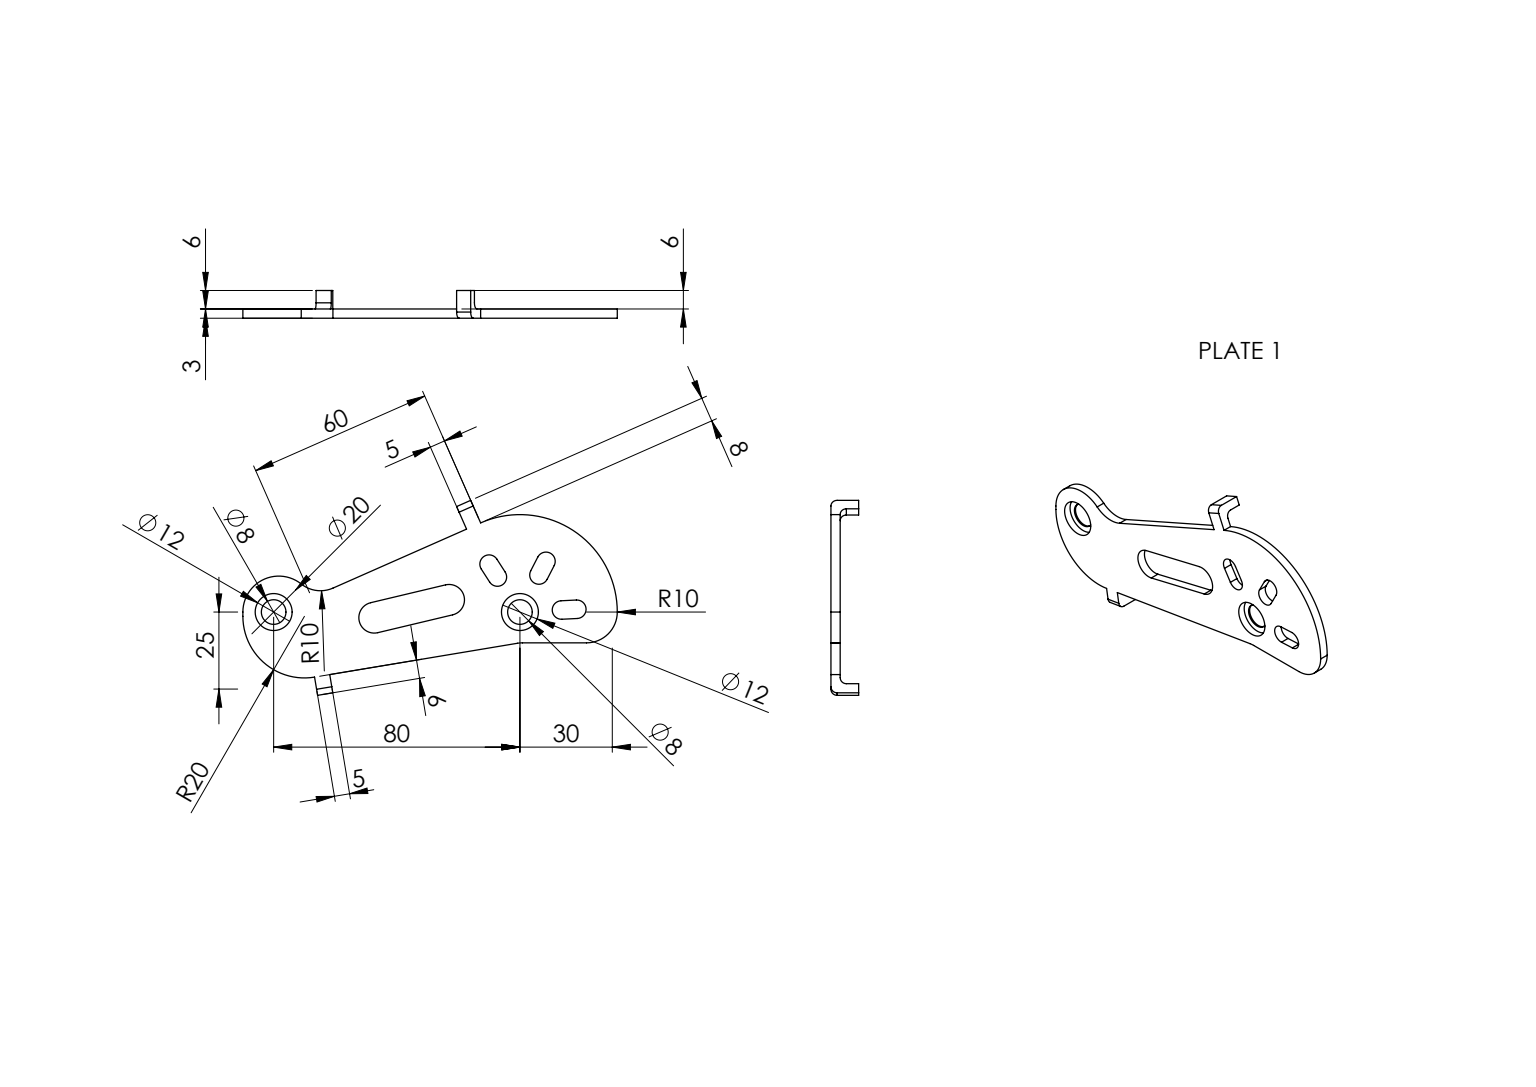
ISO-10303-21;
HEADER;
FILE_DESCRIPTION (('STEP AP214'),
    '1' );
FILE_NAME ('plate 1.step',
    '2026-10-31T03:41:51',
    ( '' ),
    ( '' ),
    'SwSTEP 2.0',
    'SolidWorks 2026',
    '' );
FILE_SCHEMA (( 'AUTOMOTIVE_DESIGN' ));
ENDSEC;

DATA;
#1=DIRECTION ( 'NONE',  ( 0.000000000000000000, 0.000000000000000000, 1.000000000000000000 ) ) ;
#5=CARTESIAN_POINT ( 'NONE',  ( 67.45386469005195806, 13.93318132202354676, 7.000000000000000000 ) ) ;
#9=ORIENTED_EDGE ( 'NONE', *, *, #4269, .F. ) ;
#17=DIRECTION ( 'NONE',  ( 1.000000000000000000, 0.000000000000000000, 0.000000000000000000 ) ) ;
#21=ORIENTED_EDGE ( 'NONE', *, *, #15147, .T. ) ;
#26=CARTESIAN_POINT ( 'NONE',  ( 101.4858053992934401, 0.9022481406819604643, 7.000000000000000000 ) ) ;
#27=DIRECTION ( 'NONE',  ( 1.000000000000000000, 0.000000000000000000, 0.000000000000000000 ) ) ;
#38=EDGE_LOOP ( 'NONE', ( #950, #5937 ) ) ;
#43=DIRECTION ( 'NONE',  ( -0.9863939238321437486, -0.1643989873053572359, 0.000000000000000000 ) ) ;
#44=CARTESIAN_POINT ( 'NONE',  ( 67.45386469005195806, 13.93318132202354676, 4.000000000000000000 ) ) ;
#50=ORIENTED_EDGE ( 'NONE', *, *, #12668, .F. ) ;
#54=ORIENTED_EDGE ( 'NONE', *, *, #8757, .F. ) ;
#57=DIRECTION ( 'NONE',  ( 0.9863939238321437486, 0.1643989873053572359, -0.000000000000000000 ) ) ;
#65=DIRECTION ( 'NONE',  ( 1.000000000000000000, 0.000000000000000000, 0.000000000000000000 ) ) ;
#76=ORIENTED_EDGE ( 'NONE', *, *, #9574, .F. ) ;
#100=CARTESIAN_POINT ( 'NONE',  ( 72.68384697807672978, 11.35494834827056110, 7.000000000000000000 ) ) ;
#101=DIRECTION ( 'NONE',  ( 0.000000000000000000, 0.000000000000000000, 1.000000000000000000 ) ) ;
#112=CYLINDRICAL_SURFACE ( 'NONE', #13936, 11.66666666666667318 ) ;
#118=CIRCLE ( 'NONE', #10455, 4.999999999999997335 ) ;
#128=EDGE_LOOP ( 'NONE', ( #4298, #9010, #776, #2710 ) ) ;
#137=CARTESIAN_POINT ( 'NONE',  ( 101.6227766016837819, 5.204170427930421283E-15, -130.1575142076926852 ) ) ;
#138=DIRECTION ( 'NONE',  ( -0.000000000000000000, -0.000000000000000000, 1.000000000000000000 ) ) ;
#151=DIRECTION ( 'NONE',  ( -0.8406209333187997235, -0.5416238976136763528, 0.000000000000000000 ) ) ;
#154=VERTEX_POINT ( 'NONE', #3488 ) ;
#169=DIRECTION ( 'NONE',  ( -0.9148936170212769170, -0.4036950204470262649, 0.000000000000000000 ) ) ;
#170=EDGE_CURVE ( 'NONE', #1510, #11203, #8177, .T. ) ;
#178=DIRECTION ( 'NONE',  ( 0.9148936170212770280, 0.4036950204470263204, -0.000000000000000000 ) ) ;
#179=DIRECTION ( 'NONE',  ( -0.9728364810787193395, -0.2314933715733012709, -0.000000000000000000 ) ) ;
#185=AXIS2_PLACEMENT_3D ( 'NONE', #6437, #12199, #1683 ) ;
#202=DIRECTION ( 'NONE',  ( -0.000000000000000000, -0.000000000000000000, -1.000000000000000000 ) ) ;
#209=VECTOR ( 'NONE', #6552, 1000.000000000000114 ) ;
#226=CIRCLE ( 'NONE', #8834, 6.000000000000005329 ) ;
#240=CARTESIAN_POINT ( 'NONE',  ( 0.000000000000000000, 0.000000000000000000, 4.500000000000000888 ) ) ;
#241=VERTEX_POINT ( 'NONE', #12080 ) ;
#257=EDGE_CURVE ( 'NONE', #8622, #3271, #11448, .T. ) ;
#261=DIRECTION ( 'NONE',  ( -2.081668171172168513E-16, 1.000000000000000000, 0.000000000000000000 ) ) ;
#265=EDGE_LOOP ( 'NONE', ( #1777, #5909, #7218, #13127 ) ) ;
#278=CYLINDRICAL_SURFACE ( 'NONE', #5273, 4.000000000000003553 ) ;
#279=ORIENTED_EDGE ( 'NONE', *, *, #14874, .F. ) ;
#287=EDGE_LOOP ( 'NONE', ( #9306, #900, #54, #10982, #12376 ) ) ;
#291=VECTOR ( 'NONE', #10020, 999.9999999999998863 ) ;
#292=VECTOR ( 'NONE', #261, 1000.000000000000000 ) ;
#303=ORIENTED_EDGE ( 'NONE', *, *, #14839, .T. ) ;
#307=LINE ( 'NONE', #10624, #1105 ) ;
#324=EDGE_LOOP ( 'NONE', ( #378, #14042, #4793, #7094 ) ) ;
#328=SURFACE_STYLE_USAGE ( .BOTH. , #10800 ) ;
#330=CIRCLE ( 'NONE', #3305, 2.999999999999988898 ) ;
#356=DIRECTION ( 'NONE',  ( 0.000000000000000000, -0.000000000000000000, -1.000000000000000000 ) ) ;
#363=ORIENTED_EDGE ( 'NONE', *, *, #14313, .F. ) ;
#370=DIRECTION ( 'NONE',  ( -0.000000000000000000, -0.000000000000000000, -1.000000000000000000 ) ) ;
#378=ORIENTED_EDGE ( 'NONE', *, *, #2401, .F. ) ;
#380=VECTOR ( 'NONE', #3922, 1000.000000000000000 ) ;
#414=VECTOR ( 'NONE', #3445, 1000.000000000000114 ) ;
#437=EDGE_CURVE ( 'NONE', #12266, #2494, #3436, .T. ) ;
#449=CARTESIAN_POINT ( 'NONE',  ( 4.000000000000000000, 4.898587196589412829E-16, 7.000000000000000000 ) ) ;
#459=CIRCLE ( 'NONE', #717, 20.00000000000000000 ) ;
#478=LINE ( 'NONE', #13313, #9423 ) ;
#497=VERTEX_POINT ( 'NONE', #5831 ) ;
#514=CARTESIAN_POINT ( 'NONE',  ( 75.20570977803312473, 12.97982004111160315, 7.000000000000000000 ) ) ;
#564=CARTESIAN_POINT ( 'NONE',  ( 101.6227766016837819, -9.999999999999994671, 4.000000000000003553 ) ) ;
#582=CARTESIAN_POINT ( 'NONE',  ( 80.00000000000000000, -9.999999999999994671, -130.1575142076926852 ) ) ;
#585=CARTESIAN_POINT ( 'NONE',  ( 83.50748565343083385, 13.38500995229612478, 7.000000000000000000 ) ) ;
#593=ADVANCED_FACE ( 'NONE', ( #8410 ), #2741, .F. ) ;
#611=DIRECTION ( 'NONE',  ( 0.9863939238321437486, 0.1643989873053572359, -0.000000000000000000 ) ) ;
#613=VERTEX_POINT ( 'NONE', #6348 ) ;
#618=ORIENTED_EDGE ( 'NONE', *, *, #1784, .F. ) ;
#619=ORIENTED_EDGE ( 'NONE', *, *, #14712, .T. ) ;
#652=DIRECTION ( 'NONE',  ( 0.9148936170212769170, 0.4036950204470262649, 0.000000000000000000 ) ) ;
#657=DIRECTION ( 'NONE',  ( -0.000000000000000000, -0.000000000000000000, -1.000000000000000000 ) ) ;
#662=ORIENTED_EDGE ( 'NONE', *, *, #2587, .T. ) ;
#665=DIRECTION ( 'NONE',  ( 0.000000000000000000, 0.000000000000000000, 1.000000000000000000 ) ) ;
#674=LINE ( 'NONE', #9057, #4725 ) ;
#693=LINE ( 'NONE', #9146, #14795 ) ;
#700=ORIENTED_EDGE ( 'NONE', *, *, #12767, .F. ) ;
#710=LINE ( 'NONE', #10011, #13396 ) ;
#715=LINE ( 'NONE', #4102, #2549 ) ;
#717=AXIS2_PLACEMENT_3D ( 'NONE', #10345, #13964, #27 ) ;
#731=EDGE_LOOP ( 'NONE', ( #12337, #9873, #12437, #11706, #9637 ) ) ;
#744=FACE_OUTER_BOUND ( 'NONE', #8998, .T. ) ;
#753=EDGE_LOOP ( 'NONE', ( #1969, #1811, #5274, #1615 ) ) ;
#758=ORIENTED_EDGE ( 'NONE', *, *, #5172, .T. ) ;
#769=DIRECTION ( 'NONE',  ( -0.9863939238321437486, -0.1643989873053574857, 0.000000000000000000 ) ) ;
#774=ORIENTED_EDGE ( 'NONE', *, *, #12921, .T. ) ;
#776=ORIENTED_EDGE ( 'NONE', *, *, #5121, .F. ) ;
#785=AXIS2_PLACEMENT_3D ( 'NONE', #4746, #10427, #14110 ) ;
#800=CARTESIAN_POINT ( 'NONE',  ( 59.43001430450886602, 34.23215029930534570, -8.169391093593850073 ) ) ;
#818=ORIENTED_EDGE ( 'NONE', *, *, #10308, .T. ) ;
#825=ORIENTED_EDGE ( 'NONE', *, *, #12060, .T. ) ;
#845=VECTOR ( 'NONE', #12005, 1000.000000000000000 ) ;
#846=VECTOR ( 'NONE', #7852, 1000.000000000000000 ) ;
#857=ADVANCED_FACE ( 'NONE', ( #3913 ), #278, .F. ) ;
#872=VECTOR ( 'NONE', #5496, 1000.000000000000000 ) ;
#873=DIRECTION ( 'NONE',  ( 0.1643989873053570416, -0.9863939238321438596, 0.000000000000000000 ) ) ;
#900=ORIENTED_EDGE ( 'NONE', *, *, #3910, .F. ) ;
#901=EDGE_CURVE ( 'NONE', #14849, #9696, #2754, .T. ) ;
#915=EDGE_CURVE ( 'NONE', #3460, #13819, #8735, .T. ) ;
#919=CARTESIAN_POINT ( 'NONE',  ( 72.68384697807672978, 11.35494834827056110, -2.000000000000000888 ) ) ;
#924=CIRCLE ( 'NONE', #3389, 2.000000000000003109 ) ;
#927=ORIENTED_EDGE ( 'NONE', *, *, #12743, .T. ) ;
#948=CARTESIAN_POINT ( 'NONE',  ( 67.23404255319148604, 28.93147646537027384, -130.1575142076926852 ) ) ;
#950=ORIENTED_EDGE ( 'NONE', *, *, #6665, .T. ) ;
#974=ORIENTED_EDGE ( 'NONE', *, *, #2510, .F. ) ;
#975=CARTESIAN_POINT ( 'NONE',  ( 31.51081190520435626, 3.030430839836910639, 4.000000000000000000 ) ) ;
#1017=SHAPE_REPRESENTATION ( 'plate 1', ( #1376 ), #2887 ) ;
#1020=EDGE_CURVE ( 'NONE', #4343, #12388, #6600, .T. ) ;
#1023=CARTESIAN_POINT ( 'NONE',  ( 10.00000000000000178, -1.390791565672601315, -130.1575142076926852 ) ) ;
#1024=PLANE ( 'NONE',  #2586 ) ;
#1043=CARTESIAN_POINT ( 'NONE',  ( 59.43001430450886602, 34.23215029930534570, -2.000000000000000000 ) ) ;
#1060=EDGE_LOOP ( 'NONE', ( #3025, #4253, #9240, #3645 ) ) ;
#1084=DIRECTION ( 'NONE',  ( 0.000000000000000000, 0.000000000000000000, 1.000000000000000000 ) ) ;
#1090=CARTESIAN_POINT ( 'NONE',  ( 33.82574562093736859, -6.697933970950280091, 7.000000000000000000 ) ) ;
#1093=EDGE_CURVE ( 'NONE', #6683, #14792, #3780, .T. ) ;
#1105=VECTOR ( 'NONE', #3625, 1000.000000000000000 ) ;
#1115=AXIS2_PLACEMENT_3D ( 'NONE', #3624, #4719, #10846 ) ;
#1127=CARTESIAN_POINT ( 'NONE',  ( 80.00000000000000000, 0.000000000000000000, 4.500000000000000888 ) ) ;
#1131=LINE ( 'NONE', #9501, #6687 ) ;
#1137=CIRCLE ( 'NONE', #7021, 3.000000000000002665 ) ;
#1142=CARTESIAN_POINT ( 'NONE',  ( 1.666666666666673624, 0.000000000000000000, -130.1575142076926852 ) ) ;
#1147=DIRECTION ( 'NONE',  ( 1.000000000000000000, 0.000000000000000000, 0.000000000000000000 ) ) ;
#1159=ORIENTED_EDGE ( 'NONE', *, *, #1020, .T. ) ;
#1166=CIRCLE ( 'NONE', #11222, 10.00000000000000000 ) ;
#1168=CIRCLE ( 'NONE', #14164, 9.999999999999994671 ) ;
#1179=ADVANCED_FACE ( 'NONE', ( #3555 ), #5032, .F. ) ;
#1181=VERTEX_POINT ( 'NONE', #1182 ) ;
#1182=CARTESIAN_POINT ( 'NONE',  ( 76.00000000000000000, 4.898587196589422689E-16, 4.500000000000003553 ) ) ;
#1191=CARTESIAN_POINT ( 'NONE',  ( 111.6227766016837961, 7.610970684806392799E-15, -130.1575142076926852 ) ) ;
#1192=CARTESIAN_POINT ( 'NONE',  ( 101.4858053992934401, 0.9022481406819604643, -2.000000000000000888 ) ) ;
#1193=ORIENTED_EDGE ( 'NONE', *, *, #15025, .F. ) ;
#1199=DIRECTION ( 'NONE',  ( -0.000000000000000000, -0.000000000000000000, 1.000000000000000000 ) ) ;
#1202=VECTOR ( 'NONE', #1786, 1000.000000000000000 ) ;
#1208=CARTESIAN_POINT ( 'NONE',  ( 88.84370878116858705, 10.64188714589527507, 7.000000000000000000 ) ) ;
#1223=EDGE_CURVE ( 'NONE', #8917, #4042, #1637, .T. ) ;
#1230=LINE ( 'NONE', #5986, #13850 ) ;
#1238=CYLINDRICAL_SURFACE ( 'NONE', #11480, 9.999999999999994671 ) ;
#1240=FACE_OUTER_BOUND ( 'NONE', #4768, .T. ) ;
#1244=ORIENTED_EDGE ( 'NONE', *, *, #9119, .F. ) ;
#1245=DIRECTION ( 'NONE',  ( -0.9863939238321437486, -0.1643989873053572359, 0.000000000000000000 ) ) ;
#1268=FACE_OUTER_BOUND ( 'NONE', #5575, .T. ) ;
#1281=CARTESIAN_POINT ( 'NONE',  ( 101.6227766016837819, -9.999999999999994671, 7.000000000000000000 ) ) ;
#1301=DIRECTION ( 'NONE',  ( -0.9863939238321436376, -0.1643989873053573192, 0.000000000000000000 ) ) ;
#1302=DIRECTION ( 'NONE',  ( -0.9863939238321437486, -0.1643989873053574857, 0.000000000000000000 ) ) ;
#1309=DIRECTION ( 'NONE',  ( 0.000000000000000000, 0.000000000000000000, 1.000000000000000000 ) ) ;
#1319=CARTESIAN_POINT ( 'NONE',  ( 19.20634328910001543, -26.21503864878155099, 4.000000000000000000 ) ) ;
#1320=ORIENTED_EDGE ( 'NONE', *, *, #13609, .F. ) ;
#1326=CIRCLE ( 'NONE', #12616, 31.62277660168379256 ) ;
#1328=ORIENTED_EDGE ( 'NONE', *, *, #3928, .F. ) ;
#1332=DIRECTION ( 'NONE',  ( -0.000000000000000000, -0.000000000000000000, 1.000000000000000000 ) ) ;
#1335=CARTESIAN_POINT ( 'NONE',  ( 80.00000000000000000, 0.000000000000000000, 4.500000000000000888 ) ) ;
#1342=DIRECTION ( 'NONE',  ( -0.000000000000000000, -0.000000000000000000, 1.000000000000000000 ) ) ;
#1353=CIRCLE ( 'NONE', #6761, 4.000000000000000000 ) ;
#1354=ORIENTED_EDGE ( 'NONE', *, *, #15079, .F. ) ;
#1358=CARTESIAN_POINT ( 'NONE',  ( 88.84370878116858705, 10.64188714589527507, -2.000000000000000888 ) ) ;
#1367=EDGE_LOOP ( 'NONE', ( #7183, #13097, #9718, #13636 ) ) ;
#1376=AXIS2_PLACEMENT_3D ( 'NONE', #7353, #6187, #9640 ) ;
#1385=DIRECTION ( 'NONE',  ( 1.000000000000000000, 0.000000000000000000, 0.000000000000000000 ) ) ;
#1396=ORIENTED_EDGE ( 'NONE', *, *, #2874, .T. ) ;
#1401=ORIENTED_EDGE ( 'NONE', *, *, #5062, .F. ) ;
#1404=CIRCLE ( 'NONE', #13462, 4.000000000000000000 ) ;
#1412=DIRECTION ( 'NONE',  ( -0.9988110320138940956, -0.04874958797097371510, 0.000000000000000000 ) ) ;
#1418=VECTOR ( 'NONE', #11737, 1000.000000000000000 ) ;
#1424=DIRECTION ( 'NONE',  ( 1.000000000000000000, 0.000000000000000000, -0.000000000000000000 ) ) ;
#1428=LINE ( 'NONE', #8483, #6858 ) ;
#1440=VECTOR ( 'NONE', #1301, 1000.000000000000114 ) ;
#1445=CARTESIAN_POINT ( 'NONE',  ( 67.23404255319145761, 28.93147646537025963, 7.000000000000000000 ) ) ;
#1452=EDGE_LOOP ( 'NONE', ( #12989, #5324, #2411, #6833, #11094 ) ) ;
#1459=EDGE_CURVE ( 'NONE', #9282, #1757, #10468, .T. ) ;
#1461=ORIENTED_EDGE ( 'NONE', *, *, #12060, .F. ) ;
#1463=ORIENTED_EDGE ( 'NONE', *, *, #915, .T. ) ;
#1468=DIRECTION ( 'NONE',  ( 0.000000000000000000, 0.000000000000000000, 1.000000000000000000 ) ) ;
#1474=ADVANCED_FACE ( 'NONE', ( #3181 ), #9091, .F. ) ;
#1475=EDGE_CURVE ( 'NONE', #7248, #11593, #5936, .T. ) ;
#1486=CARTESIAN_POINT ( 'NONE',  ( 80.00000000000000000, -9.999999999999994671, 7.000000000000000000 ) ) ;
#1489=EDGE_CURVE ( 'NONE', #12388, #13917, #12187, .T. ) ;
#1493=DIRECTION ( 'NONE',  ( -0.4036950204470279302, 0.9148936170212763619, 0.000000000000000000 ) ) ;
#1499=FACE_OUTER_BOUND ( 'NONE', #2066, .T. ) ;
#1500=LINE ( 'NONE', #12168, #14620 ) ;
#1504=VERTEX_POINT ( 'NONE', #14151 ) ;
#1505=PLANE ( 'NONE',  #15194 ) ;
#1506=CARTESIAN_POINT ( 'NONE',  ( 13.94557569532858032, -25.06424573764405395, 5.000000000000000000 ) ) ;
#1510=VERTEX_POINT ( 'NONE', #11832 ) ;
#1512=ORIENTED_EDGE ( 'NONE', *, *, #2860, .T. ) ;
#1513=FACE_OUTER_BOUND ( 'NONE', #3682, .T. ) ;
#1519=VERTEX_POINT ( 'NONE', #5 ) ;
#1521=DIRECTION ( 'NONE',  ( 0.000000000000000000, 0.000000000000000000, 1.000000000000000000 ) ) ;
#1530=LINE ( 'NONE', #9835, #380 ) ;
#1533=EDGE_LOOP ( 'NONE', ( #3960, #14213, #11513, #14850 ) ) ;
#1538=LINE ( 'NONE', #4939, #7482 ) ;
#1568=CARTESIAN_POINT ( 'NONE',  ( 85.79342132543153809, 17.83186255874426962, 4.000000000000000000 ) ) ;
#1572=PRESENTATION_STYLE_ASSIGNMENT (( #328 ) ) ;
#1576=AXIS2_PLACEMENT_3D ( 'NONE', #10565, #9261, #17 ) ;
#1578=PLANE ( 'NONE',  #2664 ) ;
#1601=DIRECTION ( 'NONE',  ( 1.000000000000000000, 0.000000000000000000, 0.000000000000000000 ) ) ;
#1610=ORIENTED_EDGE ( 'NONE', *, *, #10529, .F. ) ;
#1615=ORIENTED_EDGE ( 'NONE', *, *, #12503, .F. ) ;
#1636=EDGE_LOOP ( 'NONE', ( #8758, #1159, #8999, #4436 ) ) ;
#1637=LINE ( 'NONE', #14555, #13858 ) ;
#1646=VECTOR ( 'NONE', #5740, 1000.000000000000114 ) ;
#1653=FACE_BOUND ( 'NONE', #6790, .T. ) ;
#1658=COLOUR_RGB ( '',0.8941176470588234615, 0.8941176470588234615, 0.8941176470588234615 ) ;
#1661=DIRECTION ( 'NONE',  ( 0.000000000000000000, 0.000000000000000000, 1.000000000000000000 ) ) ;
#1668=ORIENTED_EDGE ( 'NONE', *, *, #2242, .F. ) ;
#1678=FACE_OUTER_BOUND ( 'NONE', #14305, .T. ) ;
#1679=CARTESIAN_POINT ( 'NONE',  ( 62.65957446808508280, 26.91300136313512681, -8.169391093593850073 ) ) ;
#1683=DIRECTION ( 'NONE',  ( 1.000000000000000000, 0.000000000000000000, 0.000000000000000000 ) ) ;
#1692=ORIENTED_EDGE ( 'NONE', *, *, #1093, .F. ) ;
#1700=CARTESIAN_POINT ( 'NONE',  ( 84.00000000000000000, 0.000000000000000000, 4.500000000000003553 ) ) ;
#1701=AXIS2_PLACEMENT_3D ( 'NONE', #11946, #12178, #7362 ) ;
#1708=ORIENTED_EDGE ( 'NONE', *, *, #4189, .F. ) ;
#1709=AXIS2_PLACEMENT_3D ( 'NONE', #10548, #12901, #7081 ) ;
#1711=DIRECTION ( 'NONE',  ( 0.9988110320138940956, 0.04874958797097355551, -0.000000000000000000 ) ) ;
#1717=DIRECTION ( 'NONE',  ( 0.9988110320138940956, 0.04874958797097354857, 0.000000000000000000 ) ) ;
#1721=CARTESIAN_POINT ( 'NONE',  ( 98.63205416320636232, -2.094184955359725375, 7.000000000000000000 ) ) ;
#1735=ORIENTED_EDGE ( 'NONE', *, *, #3302, .F. ) ;
#1742=VERTEX_POINT ( 'NONE', #7398 ) ;
#1752=FACE_OUTER_BOUND ( 'NONE', #12919, .T. ) ;
#1757=VERTEX_POINT ( 'NONE', #1773 ) ;
#1758=EDGE_CURVE ( 'NONE', #6683, #11986, #9775, .T. ) ;
#1763=( NAMED_UNIT ( * ) PLANE_ANGLE_UNIT ( ) SI_UNIT ( $, .RADIAN. ) );
#1771=DIRECTION ( 'NONE',  ( 0.9148936170212769170, 0.4036950204470262649, -0.000000000000000000 ) ) ;
#1773=CARTESIAN_POINT ( 'NONE',  ( 19.25177984293775069, 7.759396820770414926, 7.000000000000000000 ) ) ;
#1774=PLANE ( 'NONE',  #6975 ) ;
#1777=ORIENTED_EDGE ( 'NONE', *, *, #7772, .F. ) ;
#1784=EDGE_CURVE ( 'NONE', #2017, #6698, #6767, .T. ) ;
#1786=DIRECTION ( 'NONE',  ( 0.9863939238321437486, 0.1643989873053572359, -0.000000000000000000 ) ) ;
#1792=DIRECTION ( 'NONE',  ( 0.000000000000000000, 0.000000000000000000, 1.000000000000000000 ) ) ;
#1807=CARTESIAN_POINT ( 'NONE',  ( 75.20570977803312473, 12.97982004111159959, 4.000000000000000000 ) ) ;
#1811=ORIENTED_EDGE ( 'NONE', *, *, #7772, .T. ) ;
#1833=APPLICATION_CONTEXT ( 'automotive_design' ) ;
#1851=CYLINDRICAL_SURFACE ( 'NONE', #15082, 2.999999999999988898 ) ;
#1861=VERTEX_POINT ( 'NONE', #15066 ) ;
#1872=LINE ( 'NONE', #4418, #7681 ) ;
#1886=VECTOR ( 'NONE', #7004, 1000.000000000000000 ) ;
#1900=VECTOR ( 'NONE', #3511, 1000.000000000000000 ) ;
#1916=EDGE_CURVE ( 'NONE', #9387, #10729, #2530, .T. ) ;
#1930=DIRECTION ( 'NONE',  ( -0.9988110320138940956, -0.04874958797097371510, 0.000000000000000000 ) ) ;
#1936=LINE ( 'NONE', #4397, #846 ) ;
#1956=ADVANCED_FACE ( 'NONE', ( #5922 ), #8208, .F. ) ;
#1969=ORIENTED_EDGE ( 'NONE', *, *, #5841, .F. ) ;
#1987=DIRECTION ( 'NONE',  ( -0.000000000000000000, -0.000000000000000000, 1.000000000000000000 ) ) ;
#1993=VERTEX_POINT ( 'NONE', #9369 ) ;
#2006=CARTESIAN_POINT ( 'NONE',  ( 67.23404255319145761, 28.93147646537026318, -130.1575142076926852 ) ) ;
#2017=VERTEX_POINT ( 'NONE', #8661 ) ;
#2019=CARTESIAN_POINT ( 'NONE',  ( 8.961831343790189308, 9.104486995144789319, 4.000000000000003553 ) ) ;
#2030=DIRECTION ( 'NONE',  ( -0.000000000000000000, -0.000000000000000000, 1.000000000000000000 ) ) ;
#2046=LINE ( 'NONE', #14745, #1646 ) ;
#2052=CARTESIAN_POINT ( 'NONE',  ( 61.98919079003883326, 3.953582723775848962, 4.000000000000000000 ) ) ;
#2057=PRODUCT_DEFINITION_FORMATION_WITH_SPECIFIED_SOURCE ( 'ANY', '', #2480, .NOT_KNOWN. ) ;
#2065=LINE ( 'NONE', #6682, #14927 ) ;
#2066=EDGE_LOOP ( 'NONE', ( #2156, #3607, #7181, #7620, #5886, #1396, #303, #3086, #8875, #8957, #1193, #6098, #2265, #14266, #3257, #5444 ) ) ;
#2072=CARTESIAN_POINT ( 'NONE',  ( 18.21994936526786901, -20.29667510578869027, 4.000000000000000000 ) ) ;
#2076=VECTOR ( 'NONE', #8244, 1000.000000000000000 ) ;
#2080=ORIENTED_EDGE ( 'NONE', *, *, #12668, .T. ) ;
#2098=ORIENTED_EDGE ( 'NONE', *, *, #9330, .T. ) ;
#2107=EDGE_CURVE ( 'NONE', #14957, #4472, #1137, .T. ) ;
#2110=EDGE_LOOP ( 'NONE', ( #7467, #6376, #974, #76 ) ) ;
#2115=ORIENTED_EDGE ( 'NONE', *, *, #1223, .F. ) ;
#2121=DIRECTION ( 'NONE',  ( 0.000000000000000000, 0.000000000000000000, 1.000000000000000000 ) ) ;
#2142=VECTOR ( 'NONE', #4991, 1000.000000000000114 ) ;
#2153=FACE_OUTER_BOUND ( 'NONE', #11801, .T. ) ;
#2156=ORIENTED_EDGE ( 'NONE', *, *, #7988, .F. ) ;
#2163=EDGE_CURVE ( 'NONE', #12183, #9373, #674, .T. ) ;
#2172=AXIS2_PLACEMENT_3D ( 'NONE', #13204, #5001, #5160 ) ;
#2173=CARTESIAN_POINT ( 'NONE',  ( 18.87754531448929995, -24.24225080111726527, 7.000000000000000000 ) ) ;
#2175=DIRECTION ( 'NONE',  ( -0.9148936170212765839, -0.4036950204470271530, 0.000000000000000000 ) ) ;
#2180=AXIS2_PLACEMENT_3D ( 'NONE', #13581, #14822, #3143 ) ;
#2182=DIRECTION ( 'NONE',  ( 1.000000000000000000, 0.000000000000000000, 0.000000000000000000 ) ) ;
#2183=DIRECTION ( 'NONE',  ( 0.8406209333187990573, 0.5416238976136774630, 0.000000000000000000 ) ) ;
#2186=DIRECTION ( 'NONE',  ( 1.000000000000000000, 0.000000000000000000, 0.000000000000000000 ) ) ;
#2194=LINE ( 'NONE', #14091, #10899 ) ;
#2204=EDGE_CURVE ( 'NONE', #4704, #4042, #8972, .T. ) ;
#2227=DIRECTION ( 'NONE',  ( 0.000000000000000000, 0.000000000000000000, 1.000000000000000000 ) ) ;
#2242=EDGE_CURVE ( 'NONE', #10729, #12348, #10059, .T. ) ;
#2253=CARTESIAN_POINT ( 'NONE',  ( 80.00000000000000000, 0.000000000000000000, 4.500000000000000888 ) ) ;
#2255=VERTEX_POINT ( 'NONE', #7968 ) ;
#2265=ORIENTED_EDGE ( 'NONE', *, *, #2575, .T. ) ;
#2282=VECTOR ( 'NONE', #169, 1000.000000000000114 ) ;
#2298=DIRECTION ( 'NONE',  ( 1.000000000000000000, 0.000000000000000000, 0.000000000000000000 ) ) ;
#2313=AXIS2_PLACEMENT_3D ( 'NONE', #4662, #2489, #5948 ) ;
#2335=ADVANCED_FACE ( 'NONE', ( #5901 ), #9415, .F. ) ;
#2338=ORIENTED_EDGE ( 'NONE', *, *, #3364, .T. ) ;
#2342=AXIS2_PLACEMENT_3D ( 'NONE', #1319, #8384, #9549 ) ;
#2351=PLANE ( 'NONE',  #11505 ) ;
#2357=DIRECTION ( 'NONE',  ( 0.4571871344001383619, 0.8893705212896307888, 0.000000000000000000 ) ) ;
#2366=FACE_OUTER_BOUND ( 'NONE', #7966, .T. ) ;
#2396=EDGE_CURVE ( 'NONE', #8331, #14360, #13297, .T. ) ;
#2401=EDGE_CURVE ( 'NONE', #14060, #1181, #1131, .T. ) ;
#2402=CIRCLE ( 'NONE', #14437, 6.000000000000005329 ) ;
#2411=ORIENTED_EDGE ( 'NONE', *, *, #8973, .T. ) ;
#2449=DIRECTION ( 'NONE',  ( 1.000000000000000000, 0.000000000000000000, 0.000000000000000000 ) ) ;
#2460=ORIENTED_EDGE ( 'NONE', *, *, #11205, .F. ) ;
#2463=CARTESIAN_POINT ( 'NONE',  ( 6.000000000000000888, 0.000000000000000000, 7.000000000000000000 ) ) ;
#2469=DIRECTION ( 'NONE',  ( -0.1643989873053570416, 0.9863939238321438596, 0.000000000000000000 ) ) ;
#2471=CARTESIAN_POINT ( 'NONE',  ( 13.28797974610715116, -21.11867004231547540, 4.000000000000000000 ) ) ;
#2480=PRODUCT ( 'plate 1', 'plate 1', '', ( #7597 ) ) ;
#2489=DIRECTION ( 'NONE',  ( 0.000000000000000000, 0.000000000000000000, 1.000000000000000000 ) ) ;
#2493=ORIENTED_EDGE ( 'NONE', *, *, #4742, .F. ) ;
#2494=VERTEX_POINT ( 'NONE', #9875 ) ;
#2498=VECTOR ( 'NONE', #6820, 1000.000000000000000 ) ;
#2503=DIRECTION ( 'NONE',  ( -0.9863939238321437486, -0.1643989873053572359, 0.000000000000000000 ) ) ;
#2510=EDGE_CURVE ( 'NONE', #1861, #4961, #11576, .T. ) ;
#2521=DIRECTION ( 'NONE',  ( -0.9863939238321437486, -0.1643989873053572359, 0.000000000000000000 ) ) ;
#2530=LINE ( 'NONE', #13990, #14147 ) ;
#2539=DIRECTION ( 'NONE',  ( 1.000000000000000000, 0.000000000000000000, 0.000000000000000000 ) ) ;
#2548=VERTEX_POINT ( 'NONE', #564 ) ;
#2549=VECTOR ( 'NONE', #13472, 999.9999999999998863 ) ;
#2551=CIRCLE ( 'NONE', #4040, 3.000000000000002665 ) ;
#2557=CARTESIAN_POINT ( 'NONE',  ( 18.21994936526786901, -20.29667510578869027, 4.000000000000000000 ) ) ;
#2559=AXIS2_PLACEMENT_3D ( 'NONE', #8822, #6441, #9832 ) ;
#2562=ADVANCED_FACE ( 'NONE', ( #13330 ), #6268, .F. ) ;
#2573=CARTESIAN_POINT ( 'NONE',  ( 13.45237873341251067, -22.10506396614762537, 4.000000000000000000 ) ) ;
#2575=EDGE_CURVE ( 'NONE', #4314, #154, #2808, .T. ) ;
#2577=EDGE_CURVE ( 'NONE', #11593, #4343, #3734, .T. ) ;
#2584=VECTOR ( 'NONE', #1245, 1000.000000000000000 ) ;
#2586=AXIS2_PLACEMENT_3D ( 'NONE', #948, #4567, #6788 ) ;
#2587=EDGE_CURVE ( 'NONE', #6626, #2812, #9144, .T. ) ;
#2589=EDGE_LOOP ( 'NONE', ( #11388, #9055, #927, #8161 ) ) ;
#2590=VERTEX_POINT ( 'NONE', #1807 ) ;
#2593=CARTESIAN_POINT ( 'NONE',  ( 18.71314632718394222, -23.25585687728512241, -2.000000000000000000 ) ) ;
#2619=DIRECTION ( 'NONE',  ( 0.000000000000000000, 0.000000000000000000, 1.000000000000000000 ) ) ;
#2625=CIRCLE ( 'NONE', #6053, 1.999999999999998446 ) ;
#2631=ORIENTED_EDGE ( 'NONE', *, *, #5544, .T. ) ;
#2633=CARTESIAN_POINT ( 'NONE',  ( 70.16198417812034904, 9.730076655429538590, -2.000000000000000888 ) ) ;
#2636=ORIENTED_EDGE ( 'NONE', *, *, #2950, .F. ) ;
#2637=VECTOR ( 'NONE', #2746, 1000.000000000000000 ) ;
#2646=DIRECTION ( 'NONE',  ( 1.000000000000000000, 0.000000000000000000, 0.000000000000000000 ) ) ;
#2649=VECTOR ( 'NONE', #1199, 1000.000000000000000 ) ;
#2656=VERTEX_POINT ( 'NONE', #2964 ) ;
#2664=AXIS2_PLACEMENT_3D ( 'NONE', #12025, #5138, #7360 ) ;
#2667=PLANE ( 'NONE',  #12480 ) ;
#2668=DIRECTION ( 'NONE',  ( -1.000000000000000000, 0.000000000000000000, 0.000000000000000000 ) ) ;
#2674=ORIENTED_EDGE ( 'NONE', *, *, #1475, .F. ) ;
#2705=ORIENTED_EDGE ( 'NONE', *, *, #13390, .T. ) ;
#2709=EDGE_LOOP ( 'NONE', ( #3455, #2098 ) ) ;
#2710=ORIENTED_EDGE ( 'NONE', *, *, #12921, .F. ) ;
#2716=PRODUCT_DEFINITION_CONTEXT ( 'detailed design', #5486, 'design' ) ;
#2718=ORIENTED_EDGE ( 'NONE', *, *, #7125, .T. ) ;
#2723=LINE ( 'NONE', #2557, #9179 ) ;
#2726=EDGE_CURVE ( 'NONE', #11269, #13370, #10366, .T. ) ;
#2733=CARTESIAN_POINT ( 'NONE',  ( 0.000000000000000000, 0.000000000000000000, 7.000000000000000000 ) ) ;
#2736=CARTESIAN_POINT ( 'NONE',  ( 88.46153288930041469, 16.46030115554384565, 4.000000000000000000 ) ) ;
#2741=CYLINDRICAL_SURFACE ( 'NONE', #1701, 2.999999999999975131 ) ;
#2746=DIRECTION ( 'NONE',  ( 0.000000000000000000, 0.000000000000000000, 1.000000000000000000 ) ) ;
#2748=LINE ( 'NONE', #13340, #9757 ) ;
#2749=DIRECTION ( 'NONE',  ( -0.000000000000000000, -0.000000000000000000, 1.000000000000000000 ) ) ;
#2754=LINE ( 'NONE', #10969, #6483 ) ;
#2760=ORIENTED_EDGE ( 'NONE', *, *, #14481, .T. ) ;
#2776=EDGE_CURVE ( 'NONE', #8684, #11326, #11860, .T. ) ;
#2780=ORIENTED_EDGE ( 'NONE', *, *, #2726, .T. ) ;
#2799=EDGE_CURVE ( 'NONE', #5498, #1181, #8198, .T. ) ;
#2808=LINE ( 'NONE', #12175, #292 ) ;
#2812=VERTEX_POINT ( 'NONE', #12847 ) ;
#2817=VERTEX_POINT ( 'NONE', #12709 ) ;
#2835=DIRECTION ( 'NONE',  ( 0.5416238976136762417, -0.8406209333187996124, 0.000000000000000000 ) ) ;
#2860=EDGE_CURVE ( 'NONE', #11203, #4549, #10404, .T. ) ;
#2871=EDGE_LOOP ( 'NONE', ( #3029, #1463, #9846, #14579 ) ) ;
#2872=AXIS2_PLACEMENT_3D ( 'NONE', #1358, #14205, #14123 ) ;
#2874=EDGE_CURVE ( 'NONE', #2548, #11986, #2194, .T. ) ;
#2882=( NAMED_UNIT ( * ) SI_UNIT ( $, .STERADIAN. ) SOLID_ANGLE_UNIT ( ) );
#2883=DIRECTION ( 'NONE',  ( 0.000000000000000000, 0.000000000000000000, 1.000000000000000000 ) ) ;
#2887=( GEOMETRIC_REPRESENTATION_CONTEXT ( 3 ) GLOBAL_UNCERTAINTY_ASSIGNED_CONTEXT ( ( #8762 ) ) GLOBAL_UNIT_ASSIGNED_CONTEXT ( ( #5206, #8711, #2882 ) ) REPRESENTATION_CONTEXT ( 'NONE', 'WORKASPACE' ) );
#2892=VECTOR ( 'NONE', #14504, 1000.000000000000000 ) ;
#2896=ORIENTED_EDGE ( 'NONE', *, *, #14272, .T. ) ;
#2919=ADVANCED_FACE ( 'NONE', ( #9558 ), #1851, .F. ) ;
#2920=CARTESIAN_POINT ( 'NONE',  ( -4.000000000000000000, 0.000000000000000000, 4.500000000000000888 ) ) ;
#2930=CARTESIAN_POINT ( 'NONE',  ( 64.00448238961524794, 36.25062540154047497, 5.000000000000000888 ) ) ;
#2942=CARTESIAN_POINT ( 'NONE',  ( 19.20634328910001543, -26.21503864878155099, -2.000000000000000000 ) ) ;
#2949=CARTESIAN_POINT ( 'NONE',  ( 84.00000000000000000, 0.000000000000000000, 4.000000000000003553 ) ) ;
#2950=EDGE_CURVE ( 'NONE', #4042, #11203, #2551, .T. ) ;
#2964=CARTESIAN_POINT ( 'NONE',  ( 59.43001430450886602, 34.23215029930534570, 5.000000000000000888 ) ) ;
#2967=EDGE_CURVE ( 'NONE', #11474, #10155, #7711, .T. ) ;
#2969=ORIENTED_EDGE ( 'NONE', *, *, #2776, .F. ) ;
#2972=DIRECTION ( 'NONE',  ( 0.1643989873053574302, -0.9863939238321437486, 0.000000000000000000 ) ) ;
#2980=ADVANCED_FACE ( 'NONE', ( #3004 ), #1774, .F. ) ;
#2992=CARTESIAN_POINT ( 'NONE',  ( 6.000000000000000888, 0.000000000000000000, 4.500000000000000888 ) ) ;
#2998=EDGE_CURVE ( 'NONE', #4961, #5235, #11224, .T. ) ;
#3004=FACE_OUTER_BOUND ( 'NONE', #3852, .T. ) ;
#3016=LINE ( 'NONE', #2942, #5641 ) ;
#3022=DIRECTION ( 'NONE',  ( 0.000000000000000000, 0.000000000000000000, 1.000000000000000000 ) ) ;
#3025=ORIENTED_EDGE ( 'NONE', *, *, #3209, .T. ) ;
#3028=EDGE_LOOP ( 'NONE', ( #10679, #15182, #11673, #9697 ) ) ;
#3029=ORIENTED_EDGE ( 'NONE', *, *, #8709, .F. ) ;
#3030=CARTESIAN_POINT ( 'NONE',  ( 88.46153288930041469, 16.46030115554384565, 7.000000000000000000 ) ) ;
#3038=DIRECTION ( 'NONE',  ( 0.4036950204470263204, -0.9148936170212770280, 0.000000000000000000 ) ) ;
#3040=ORIENTED_EDGE ( 'NONE', *, *, #2967, .T. ) ;
#3041=DIRECTION ( 'NONE',  ( 0.5416238976136762417, -0.8406209333187997235, -0.000000000000000000 ) ) ;
#3048=ADVANCED_FACE ( 'NONE', ( #13603 ), #3085, .F. ) ;
#3085=CYLINDRICAL_SURFACE ( 'NONE', #9180, 6.000000000000000888 ) ;
#3086=ORIENTED_EDGE ( 'NONE', *, *, #9173, .T. ) ;
#3097=EDGE_CURVE ( 'NONE', #9387, #12669, #1936, .T. ) ;
#3104=CARTESIAN_POINT ( 'NONE',  ( 86.17559721729969624, 12.01344854909570259, 4.000000000000000000 ) ) ;
#3108=CARTESIAN_POINT ( 'NONE',  ( 93.34550147531103903, 3.654933296868752457, -2.000000000000000888 ) ) ;
#3124=DIRECTION ( 'NONE',  ( 0.1643989873053578465, -0.9863939238321436376, 0.000000000000000000 ) ) ;
#3143=DIRECTION ( 'NONE',  ( -0.4571871344001417481, -0.8893705212896291235, 0.000000000000000000 ) ) ;
#3164=ORIENTED_EDGE ( 'NONE', *, *, #9841, .T. ) ;
#3172=VERTEX_POINT ( 'NONE', #7995 ) ;
#3181=FACE_OUTER_BOUND ( 'NONE', #5045, .T. ) ;
#3209=EDGE_CURVE ( 'NONE', #4384, #13626, #1230, .T. ) ;
#3221=CARTESIAN_POINT ( 'NONE',  ( 74.00000000000000000, 7.347880794884117764E-16, 4.500000000000000888 ) ) ;
#3222=ORIENTED_EDGE ( 'NONE', *, *, #10042, .T. ) ;
#3242=VERTEX_POINT ( 'NONE', #2463 ) ;
#3249=ORIENTED_EDGE ( 'NONE', *, *, #10369, .F. ) ;
#3255=DIRECTION ( 'NONE',  ( -1.000000000000000000, 0.000000000000000000, 0.000000000000000000 ) ) ;
#3256=CARTESIAN_POINT ( 'NONE',  ( 69.97572749000833880, 15.55805301486455683, 7.000000000000000000 ) ) ;
#3257=ORIENTED_EDGE ( 'NONE', *, *, #13814, .T. ) ;
#3261=EDGE_CURVE ( 'NONE', #1993, #8917, #12384, .T. ) ;
#3271=VERTEX_POINT ( 'NONE', #10537 ) ;
#3272=CARTESIAN_POINT ( 'NONE',  ( 61.98919079003883326, 3.953582723775848962, 7.000000000000000000 ) ) ;
#3273=DIRECTION ( 'NONE',  ( 0.4036950204470283188, -0.9148936170212761398, -0.000000000000000000 ) ) ;
#3290=ORIENTED_EDGE ( 'NONE', *, *, #7125, .F. ) ;
#3292=VERTEX_POINT ( 'NONE', #12818 ) ;
#3294=CARTESIAN_POINT ( 'NONE',  ( 80.00000000000000000, 0.000000000000000000, 4.500000000000003553 ) ) ;
#3300=CARTESIAN_POINT ( 'NONE',  ( 66.02295749185037721, 31.67615731643408949, 4.000000000000000000 ) ) ;
#3302=EDGE_CURVE ( 'NONE', #3709, #8012, #6990, .T. ) ;
#3305=AXIS2_PLACEMENT_3D ( 'NONE', #3104, #1792, #11316 ) ;
#3330=DIRECTION ( 'NONE',  ( 0.000000000000000000, 0.000000000000000000, 1.000000000000000000 ) ) ;
#3334=FACE_OUTER_BOUND ( 'NONE', #753, .T. ) ;
#3352=DIRECTION ( 'NONE',  ( -0.4036950204470285408, 0.9148936170212760288, 0.000000000000000000 ) ) ;
#3364=EDGE_CURVE ( 'NONE', #8684, #5234, #9894, .T. ) ;
#3365=EDGE_CURVE ( 'NONE', #2017, #7876, #9196, .T. ) ;
#3368=CARTESIAN_POINT ( 'NONE',  ( 58.14665764790533586, -0.9105996816177489572, 7.000000000000000000 ) ) ;
#3370=ORIENTED_EDGE ( 'NONE', *, *, #8629, .T. ) ;
#3371=CIRCLE ( 'NONE', #11691, 3.000000000000002665 ) ;
#3389=AXIS2_PLACEMENT_3D ( 'NONE', #4691, #10814, #4989 ) ;
#3399=DIRECTION ( 'NONE',  ( 1.000000000000000000, 0.000000000000000000, 0.000000000000000000 ) ) ;
#3400=DIRECTION ( 'NONE',  ( 1.000000000000000000, 0.000000000000000000, 0.000000000000000000 ) ) ;
#3408=FACE_OUTER_BOUND ( 'NONE', #9800, .T. ) ;
#3409=DIRECTION ( 'NONE',  ( 0.000000000000000000, 0.000000000000000000, 1.000000000000000000 ) ) ;
#3413=CARTESIAN_POINT ( 'NONE',  ( 80.00000000000000000, 0.000000000000000000, -130.1575142076926852 ) ) ;
#3425=CARTESIAN_POINT ( 'NONE',  ( 66.02295749185039142, 31.67615731643408949, 2.000000000000000000 ) ) ;
#3433=ORIENTED_EDGE ( 'NONE', *, *, #5924, .T. ) ;
#3436=LINE ( 'NONE', #1208, #3855 ) ;
#3444=CARTESIAN_POINT ( 'NONE',  ( 59.43001430450886602, 34.23215029930534570, -8.169391093593850073 ) ) ;
#3445=DIRECTION ( 'NONE',  ( -0.5416238976136773520, 0.8406209333187989463, 0.000000000000000000 ) ) ;
#3448=DIRECTION ( 'NONE',  ( -0.000000000000000000, -0.000000000000000000, 1.000000000000000000 ) ) ;
#3455=ORIENTED_EDGE ( 'NONE', *, *, #15119, .T. ) ;
#3460=VERTEX_POINT ( 'NONE', #3221 ) ;
#3461=VERTEX_POINT ( 'NONE', #12516 ) ;
#3465=DIRECTION ( 'NONE',  ( 0.9988110320138940956, 0.04874958797097355551, 0.000000000000000000 ) ) ;
#3488=CARTESIAN_POINT ( 'NONE',  ( -9.999999999999998224, 0.000000000000000000, 4.000000000000003553 ) ) ;
#3494=CARTESIAN_POINT ( 'NONE',  ( 65.21556745095632834, 33.50594455047664866, -2.000000000000000000 ) ) ;
#3495=DIRECTION ( 'NONE',  ( -0.000000000000000000, -0.000000000000000000, 1.000000000000000000 ) ) ;
#3503=VECTOR ( 'NONE', #13162, 1000.000000000000000 ) ;
#3507=VERTEX_POINT ( 'NONE', #5529 ) ;
#3511=DIRECTION ( 'NONE',  ( 0.000000000000000000, 0.000000000000000000, 1.000000000000000000 ) ) ;
#3523=CARTESIAN_POINT ( 'NONE',  ( 67.23404255319148604, 28.93147646537027384, 4.000000000000003553 ) ) ;
#3525=EDGE_CURVE ( 'NONE', #3993, #3242, #3858, .T. ) ;
#3526=ORIENTED_EDGE ( 'NONE', *, *, #15119, .F. ) ;
#3542=VECTOR ( 'NONE', #2175, 1000.000000000000000 ) ;
#3552=AXIS2_PLACEMENT_3D ( 'NONE', #3800, #13014, #10801 ) ;
#3555=FACE_OUTER_BOUND ( 'NONE', #12397, .T. ) ;
#3560=DIRECTION ( 'NONE',  ( -1.000000000000000000, 0.000000000000000000, 0.000000000000000000 ) ) ;
#3561=ORIENTED_EDGE ( 'NONE', *, *, #15147, .F. ) ;
#3568=ORIENTED_EDGE ( 'NONE', *, *, #4269, .T. ) ;
#3570=CARTESIAN_POINT ( 'NONE',  ( 31.51081190520435626, 3.030430839836910639, 7.000000000000000000 ) ) ;
#3594=ORIENTED_EDGE ( 'NONE', *, *, #14695, .T. ) ;
#3607=ORIENTED_EDGE ( 'NONE', *, *, #14874, .T. ) ;
#3613=FACE_OUTER_BOUND ( 'NONE', #10521, .T. ) ;
#3624=CARTESIAN_POINT ( 'NONE',  ( 32.66827876307085887, -1.833751565556681173, 4.000000000000000000 ) ) ;
#3625=DIRECTION ( 'NONE',  ( -0.000000000000000000, -0.000000000000000000, -1.000000000000000000 ) ) ;
#3634=DIRECTION ( 'NONE',  ( 0.9728364810787193395, 0.2314933715733012431, 0.000000000000000000 ) ) ;
#3645=ORIENTED_EDGE ( 'NONE', *, *, #5172, .F. ) ;
#3648=FACE_BOUND ( 'NONE', #287, .T. ) ;
#3660=DIRECTION ( 'NONE',  ( 0.000000000000000000, 0.000000000000000000, 1.000000000000000000 ) ) ;
#3681=DIRECTION ( 'NONE',  ( 1.000000000000000000, 0.000000000000000000, 0.000000000000000000 ) ) ;
#3682=EDGE_LOOP ( 'NONE', ( #8348, #1401, #8006, #12251 ) ) ;
#3693=CARTESIAN_POINT ( 'NONE',  ( 31.51081190520435626, 3.030430839836910639, -2.000000000000000888 ) ) ;
#3709=VERTEX_POINT ( 'NONE', #11035 ) ;
#3728=FACE_OUTER_BOUND ( 'NONE', #3813, .T. ) ;
#3733=AXIS2_PLACEMENT_3D ( 'NONE', #2072, #769, #6763 ) ;
#3734=CIRCLE ( 'NONE', #4980, 4.999999999999997335 ) ;
#3741=CARTESIAN_POINT ( 'NONE',  ( 93.49175023922396122, 0.6585002008270834928, -2.000000000000000888 ) ) ;
#3747=CARTESIAN_POINT ( 'NONE',  ( 0.000000000000000000, 0.000000000000000000, 4.500000000000000888 ) ) ;
#3753=CARTESIAN_POINT ( 'NONE',  ( 93.49175023922396122, 0.6585002008270834928, 7.000000000000000000 ) ) ;
#3756=ORIENTED_EDGE ( 'NONE', *, *, #5136, .T. ) ;
#3760=LINE ( 'NONE', #12981, #13183 ) ;
#3761=DIRECTION ( 'NONE',  ( -0.9148936170212769170, -0.4036950204470262649, 0.000000000000000000 ) ) ;
#3762=CARTESIAN_POINT ( 'NONE',  ( 86.17559721729969624, 12.01344854909570259, -2.000000000000000888 ) ) ;
#3776=AXIS2_PLACEMENT_3D ( 'NONE', #7622, #14248, #7254 ) ;
#3780=LINE ( 'NONE', #1486, #4029 ) ;
#3785=CARTESIAN_POINT ( 'NONE',  ( 98.48580539929344013, 0.9022481406819604643, 7.000000000000000000 ) ) ;
#3789=DIRECTION ( 'NONE',  ( 0.1643989873053573469, -0.9863939238321437486, 0.000000000000000000 ) ) ;
#3795=ORIENTED_EDGE ( 'NONE', *, *, #14182, .F. ) ;
#3796=FACE_BOUND ( 'NONE', #14928, .T. ) ;
#3800=CARTESIAN_POINT ( 'NONE',  ( 80.82762530298222714, -19.99999999999999645, 7.000000000000006217 ) ) ;
#3808=AXIS2_PLACEMENT_3D ( 'NONE', #9493, #8260, #8404 ) ;
#3813=EDGE_LOOP ( 'NONE', ( #12460, #13499, #4147, #618, #1610, #12136, #15055, #4610 ) ) ;
#3814=EDGE_CURVE ( 'NONE', #154, #6827, #9014, .T. ) ;
#3816=LINE ( 'NONE', #12031, #2637 ) ;
#3824=DIRECTION ( 'NONE',  ( 0.000000000000000000, 0.000000000000000000, 1.000000000000000000 ) ) ;
#3828=ORIENTED_EDGE ( 'NONE', *, *, #11609, .T. ) ;
#3841=CARTESIAN_POINT ( 'NONE',  ( 13.78117670802322259, -24.07785181381190753, 2.000000000000000000 ) ) ;
#3843=DIRECTION ( 'NONE',  ( 0.1643989873053574580, -0.9863939238321436376, 0.000000000000000000 ) ) ;
#3844=DIRECTION ( 'NONE',  ( 0.000000000000000000, 0.000000000000000000, 1.000000000000000000 ) ) ;
#3852=EDGE_LOOP ( 'NONE', ( #9445, #13967, #50, #8954 ) ) ;
#3855=VECTOR ( 'NONE', #2357, 1000.000000000000114 ) ;
#3858=CIRCLE ( 'NONE', #11937, 6.000000000000000888 ) ;
#3869=CARTESIAN_POINT ( 'NONE',  ( 69.97572749000833880, 15.55805301486455683, -2.000000000000000888 ) ) ;
#3883=ORIENTED_EDGE ( 'NONE', *, *, #11255, .F. ) ;
#3884=FACE_BOUND ( 'NONE', #2709, .T. ) ;
#3886=( LENGTH_UNIT ( ) NAMED_UNIT ( * ) SI_UNIT ( .MILLI., .METRE. ) );
#3890=CIRCLE ( 'NONE', #6594, 2.999999999999975131 ) ;
#3891=AXIS2_PLACEMENT_3D ( 'NONE', #14427, #3893, #9874 ) ;
#3893=DIRECTION ( 'NONE',  ( -1.000000000000000000, -2.081668171172168513E-16, 0.000000000000000000 ) ) ;
#3894=DIRECTION ( 'NONE',  ( 0.1643989873053578465, -0.9863939238321436376, 0.000000000000000000 ) ) ;
#3905=DIRECTION ( 'NONE',  ( 1.000000000000000000, 0.000000000000000000, 0.000000000000000000 ) ) ;
#3910=EDGE_CURVE ( 'NONE', #1519, #5234, #9115, .T. ) ;
#3913=FACE_OUTER_BOUND ( 'NONE', #13789, .T. ) ;
#3922=DIRECTION ( 'NONE',  ( 0.000000000000000000, 0.000000000000000000, 1.000000000000000000 ) ) ;
#3928=EDGE_CURVE ( 'NONE', #1504, #7876, #11846, .T. ) ;
#3943=PLANE ( 'NONE',  #5050 ) ;
#3950=ORIENTED_EDGE ( 'NONE', *, *, #15174, .T. ) ;
#3960=ORIENTED_EDGE ( 'NONE', *, *, #4941, .F. ) ;
#3980=CARTESIAN_POINT ( 'NONE',  ( 18.71314632718394222, -23.25585687728512241, -2.000000000000000000 ) ) ;
#3981=DIRECTION ( 'NONE',  ( 0.000000000000000000, -1.000000000000000000, 0.000000000000000000 ) ) ;
#3993=VERTEX_POINT ( 'NONE', #8329 ) ;
#3998=DIRECTION ( 'NONE',  ( 0.4571871344001385284, 0.8893705212896308998, -0.000000000000000000 ) ) ;
#4008=VERTEX_POINT ( 'NONE', #10714 ) ;
#4012=EDGE_CURVE ( 'NONE', #3271, #497, #7178, .T. ) ;
#4029=VECTOR ( 'NONE', #8322, 1000.000000000000000 ) ;
#4033=FACE_BOUND ( 'NONE', #15004, .T. ) ;
#4039=DIRECTION ( 'NONE',  ( 1.000000000000000000, 0.000000000000000000, 0.000000000000000000 ) ) ;
#4040=AXIS2_PLACEMENT_3D ( 'NONE', #3785, #8763, #2646 ) ;
#4042=VERTEX_POINT ( 'NONE', #1721 ) ;
#4044=DIRECTION ( 'NONE',  ( 0.000000000000000000, 0.000000000000000000, 1.000000000000000000 ) ) ;
#4052=ORIENTED_EDGE ( 'NONE', *, *, #170, .T. ) ;
#4055=CARTESIAN_POINT ( 'NONE',  ( 13.28797974610715116, -21.11867004231547540, 7.000000000000000000 ) ) ;
#4063=DIRECTION ( 'NONE',  ( -0.4571871344001416926, -0.8893705212896291235, -0.000000000000000000 ) ) ;
#4064=DIRECTION ( 'NONE',  ( 0.000000000000000000, 0.000000000000000000, 1.000000000000000000 ) ) ;
#4068=DIRECTION ( 'NONE',  ( -0.000000000000000000, -0.000000000000000000, 1.000000000000000000 ) ) ;
#4070=ORIENTED_EDGE ( 'NONE', *, *, #2107, .F. ) ;
#4090=DIRECTION ( 'NONE',  ( 0.9728364810787193395, 0.2314933715733012709, 0.000000000000000000 ) ) ;
#4097=VECTOR ( 'NONE', #7107, 1000.000000000000000 ) ;
#4101=DIRECTION ( 'NONE',  ( 0.000000000000000000, 0.000000000000000000, 1.000000000000000000 ) ) ;
#4102=CARTESIAN_POINT ( 'NONE',  ( 62.65957446808508280, 26.91300136313512681, 4.000000000000000000 ) ) ;
#4121=DIRECTION ( 'NONE',  ( 0.000000000000000000, 0.000000000000000000, 1.000000000000000000 ) ) ;
#4122=VECTOR ( 'NONE', #13651, 1000.000000000000000 ) ;
#4127=VECTOR ( 'NONE', #3022, 1000.000000000000000 ) ;
#4128=ORIENTED_EDGE ( 'NONE', *, *, #12202, .F. ) ;
#4131=ADVANCED_FACE ( 'NONE', ( #12079 ), #5120, .T. ) ;
#4133=EDGE_CURVE ( 'NONE', #7876, #2548, #8903, .T. ) ;
#4140=DIRECTION ( 'NONE',  ( 1.000000000000000000, 0.000000000000000000, 0.000000000000000000 ) ) ;
#4141=AXIS2_PLACEMENT_3D ( 'NONE', #10799, #12166, #9803 ) ;
#4147=ORIENTED_EDGE ( 'NONE', *, *, #14712, .F. ) ;
#4154=DIRECTION ( 'NONE',  ( 0.000000000000000000, 0.000000000000000000, 1.000000000000000000 ) ) ;
#4168=ORIENTED_EDGE ( 'NONE', *, *, #11858, .T. ) ;
#4176=DIRECTION ( 'NONE',  ( 0.2314933715733012709, -0.9728364810787193395, 0.000000000000000000 ) ) ;
#4189=EDGE_CURVE ( 'NONE', #7258, #13917, #8471, .T. ) ;
#4208=ORIENTED_EDGE ( 'NONE', *, *, #7877, .T. ) ;
#4214=CARTESIAN_POINT ( 'NONE',  ( 79.18363542992865689, -10.13606076167855541, 4.000000000000003553 ) ) ;
#4221=CARTESIAN_POINT ( 'NONE',  ( 0.000000000000000000, 0.000000000000000000, 7.000000000000000000 ) ) ;
#4232=CARTESIAN_POINT ( 'NONE',  ( 67.23404255319145761, 28.93147646537025963, 4.000000000000000000 ) ) ;
#4240=EDGE_CURVE ( 'NONE', #11326, #7126, #1872, .T. ) ;
#4246=ORIENTED_EDGE ( 'NONE', *, *, #4012, .T. ) ;
#4252=DIRECTION ( 'NONE',  ( 0.000000000000000000, 0.000000000000000000, 1.000000000000000000 ) ) ;
#4253=ORIENTED_EDGE ( 'NONE', *, *, #9574, .T. ) ;
#4260=DIRECTION ( 'NONE',  ( 0.000000000000000000, 0.000000000000000000, 1.000000000000000000 ) ) ;
#4269=EDGE_CURVE ( 'NONE', #9282, #497, #10165, .T. ) ;
#4278=CARTESIAN_POINT ( 'NONE',  ( 58.14665764790533586, -0.9105996816177498454, 4.000000000000000000 ) ) ;
#4284=CARTESIAN_POINT ( 'NONE',  ( 32.66827876307085887, -1.833751565556681173, -2.000000000000000888 ) ) ;
#4293=EDGE_CURVE ( 'NONE', #14530, #10918, #9016, .T. ) ;
#4298=ORIENTED_EDGE ( 'NONE', *, *, #1475, .T. ) ;
#4305=CIRCLE ( 'NONE', #5779, 2.000000000000000000 ) ;
#4308=CIRCLE ( 'NONE', #14117, 6.000000000000005329 ) ;
#4311=VERTEX_POINT ( 'NONE', #2949 ) ;
#4314=VERTEX_POINT ( 'NONE', #13778 ) ;
#4315=CIRCLE ( 'NONE', #3808, 2.999999999999988898 ) ;
#4336=CARTESIAN_POINT ( 'NONE',  ( -4.000000000000000000, 0.000000000000000000, 7.000000000000000000 ) ) ;
#4343=VERTEX_POINT ( 'NONE', #1090 ) ;
#4351=CIRCLE ( 'NONE', #13671, 9.999999999999994671 ) ;
#4369=ORIENTED_EDGE ( 'NONE', *, *, #10988, .F. ) ;
#4380=ORIENTED_EDGE ( 'NONE', *, *, #6087, .T. ) ;
#4384=VERTEX_POINT ( 'NONE', #13929 ) ;
#4385=CARTESIAN_POINT ( 'NONE',  ( 83.50748565343083385, 13.38500995229612478, 4.000000000000000000 ) ) ;
#4397=CARTESIAN_POINT ( 'NONE',  ( 65.21556745095632834, 33.50594455047664866, -2.000000000000000000 ) ) ;
#4418=CARTESIAN_POINT ( 'NONE',  ( 75.68384697807671557, 11.35494834827056110, -2.000000000000000888 ) ) ;
#4423=ORIENTED_EDGE ( 'NONE', *, *, #1489, .F. ) ;
#4436=ORIENTED_EDGE ( 'NONE', *, *, #8997, .F. ) ;
#4438=PLANE ( 'NONE',  #4862 ) ;
#4440=EDGE_CURVE ( 'NONE', #2255, #14957, #693, .T. ) ;
#4441=CYLINDRICAL_SURFACE ( 'NONE', #9972, 4.999999999999997335 ) ;
#4451=ADVANCED_FACE ( 'NONE', ( #10300 ), #13827, .F. ) ;
#4459=DIRECTION ( 'NONE',  ( 1.000000000000000000, 0.000000000000000000, 0.000000000000000000 ) ) ;
#4472=VERTEX_POINT ( 'NONE', #13681 ) ;
#4477=FACE_OUTER_BOUND ( 'NONE', #6462, .T. ) ;
#4489=CARTESIAN_POINT ( 'NONE',  ( 80.82762530298222714, -19.99999999999999645, -130.1575142076926852 ) ) ;
#4490=DIRECTION ( 'NONE',  ( 0.000000000000000000, 0.000000000000000000, 1.000000000000000000 ) ) ;
#4496=ADVANCED_FACE ( 'NONE', ( #2153 ), #14999, .F. ) ;
#4504=ORIENTED_EDGE ( 'NONE', *, *, #1093, .T. ) ;
#4509=EDGE_CURVE ( 'NONE', #11060, #5604, #13034, .T. ) ;
#4534=DIRECTION ( 'NONE',  ( -0.000000000000000000, -0.000000000000000000, 1.000000000000000000 ) ) ;
#4537=DIRECTION ( 'NONE',  ( -0.000000000000000000, -0.000000000000000000, 1.000000000000000000 ) ) ;
#4549=VERTEX_POINT ( 'NONE', #7137 ) ;
#4565=CARTESIAN_POINT ( 'NONE',  ( 60.64109936584995353, 31.48746944824151583, 2.000000000000000000 ) ) ;
#4567=DIRECTION ( 'NONE',  ( -0.4036950204470272086, 0.9148936170212765839, 0.000000000000000000 ) ) ;
#4587=EDGE_CURVE ( 'NONE', #4311, #5498, #11619, .T. ) ;
#4596=AXIS2_PLACEMENT_3D ( 'NONE', #13128, #57, #2469 ) ;
#4610=ORIENTED_EDGE ( 'NONE', *, *, #1916, .T. ) ;
#4621=CARTESIAN_POINT ( 'NONE',  ( 84.00000000000000000, 0.000000000000000000, -130.1575142076926852 ) ) ;
#4626=DIRECTION ( 'NONE',  ( -0.000000000000000000, -0.000000000000000000, 1.000000000000000000 ) ) ;
#4662=CARTESIAN_POINT ( 'NONE',  ( 72.68384697807672978, 11.35494834827056110, 4.000000000000000000 ) ) ;
#4665=EDGE_CURVE ( 'NONE', #8012, #9282, #14444, .T. ) ;
#4670=DIRECTION ( 'NONE',  ( -0.4036950204470279302, 0.9148936170212763619, 0.000000000000000000 ) ) ;
#4691=CARTESIAN_POINT ( 'NONE',  ( 60.23740434540291488, 32.40236306526279009, 5.000000000000000888 ) ) ;
#4692=LINE ( 'NONE', #2593, #10492 ) ;
#4696=FACE_OUTER_BOUND ( 'NONE', #10904, .T. ) ;
#4699=ADVANCED_FACE ( 'NONE', ( #1678 ), #7521, .T. ) ;
#4704=VERTEX_POINT ( 'NONE', #12110 ) ;
#4719=DIRECTION ( 'NONE',  ( 0.000000000000000000, 0.000000000000000000, 1.000000000000000000 ) ) ;
#4720=PLANE ( 'NONE',  #9221 ) ;
#4725=VECTOR ( 'NONE', #6743, 1000.000000000000114 ) ;
#4737=DIRECTION ( 'NONE',  ( -0.000000000000000000, -0.000000000000000000, 1.000000000000000000 ) ) ;
#4742=EDGE_CURVE ( 'NONE', #4311, #14060, #15049, .T. ) ;
#4746=CARTESIAN_POINT ( 'NONE',  ( 80.00000000000000000, 0.000000000000000000, 4.500000000000000888 ) ) ;
#4766=ADVANCED_FACE ( 'NONE', ( #5154 ), #14519, .F. ) ;
#4768=EDGE_LOOP ( 'NONE', ( #8741, #14497, #9548, #6568 ) ) ;
#4775=FACE_OUTER_BOUND ( 'NONE', #2110, .T. ) ;
#4793=ORIENTED_EDGE ( 'NONE', *, *, #4587, .T. ) ;
#4817=LINE ( 'NONE', #14188, #8462 ) ;
#4818=LINE ( 'NONE', #5341, #209 ) ;
#4823=DIRECTION ( 'NONE',  ( 0.000000000000000000, 0.000000000000000000, 1.000000000000000000 ) ) ;
#4824=DIRECTION ( 'NONE',  ( 1.000000000000000000, 0.000000000000000000, 0.000000000000000000 ) ) ;
#4835=AXIS2_PLACEMENT_3D ( 'NONE', #11018, #7489, #1493 ) ;
#4846=DIRECTION ( 'NONE',  ( 0.000000000000000000, 0.000000000000000000, 1.000000000000000000 ) ) ;
#4862=AXIS2_PLACEMENT_3D ( 'NONE', #10046, #14743, #9121 ) ;
#4864=VERTEX_POINT ( 'NONE', #4214 ) ;
#4892=ORIENTED_EDGE ( 'NONE', *, *, #7393, .T. ) ;
#4899=DIRECTION ( 'NONE',  ( 1.000000000000000000, 0.000000000000000000, 0.000000000000000000 ) ) ;
#4907=DIRECTION ( 'NONE',  ( 1.000000000000000000, 0.000000000000000000, 0.000000000000000000 ) ) ;
#4921=DIRECTION ( 'NONE',  ( -1.000000000000000000, 0.000000000000000000, 0.000000000000000000 ) ) ;
#4925=CIRCLE ( 'NONE', #13500, 6.000000000000000888 ) ;
#4938=PLANE ( 'NONE',  #10993 ) ;
#4939=CARTESIAN_POINT ( 'NONE',  ( 93.34550147531103903, 3.654933296868752457, 7.000000000000000000 ) ) ;
#4941=EDGE_CURVE ( 'NONE', #9696, #4314, #459, .T. ) ;
#4942=CYLINDRICAL_SURFACE ( 'NONE', #1709, 2.000000000000000444 ) ;
#4956=CARTESIAN_POINT ( 'NONE',  ( 111.6227766016837961, 7.610970684806392799E-15, 4.000000000000003553 ) ) ;
#4957=EDGE_CURVE ( 'NONE', #4704, #1510, #9544, .T. ) ;
#4961=VERTEX_POINT ( 'NONE', #10422 ) ;
#4975=DIRECTION ( 'NONE',  ( -0.4036950204470267645, 0.9148936170212768060, 0.000000000000000000 ) ) ;
#4980=AXIS2_PLACEMENT_3D ( 'NONE', #7361, #1661, #11033 ) ;
#4982=ADVANCED_FACE ( 'NONE', ( #13880 ), #2351, .F. ) ;
#4989=DIRECTION ( 'NONE',  ( -0.4036950204470279302, 0.9148936170212763619, 1.734723475976804333E-15 ) ) ;
#4991=DIRECTION ( 'NONE',  ( -0.4036950204470267645, 0.9148936170212768060, 0.000000000000000000 ) ) ;
#4997=DIRECTION ( 'NONE',  ( 1.000000000000000000, 0.000000000000000000, 0.000000000000000000 ) ) ;
#5001=DIRECTION ( 'NONE',  ( -0.000000000000000000, -0.000000000000000000, -1.000000000000000000 ) ) ;
#5005=LINE ( 'NONE', #14457, #14893 ) ;
#5023=DIRECTION ( 'NONE',  ( 0.5416238976136762417, -0.8406209333187996124, 0.000000000000000000 ) ) ;
#5026=ORIENTED_EDGE ( 'NONE', *, *, #13760, .T. ) ;
#5032=CYLINDRICAL_SURFACE ( 'NONE', #11394, 2.999999999999988898 ) ;
#5045=EDGE_LOOP ( 'NONE', ( #758, #13167, #6781, #1244 ) ) ;
#5050=AXIS2_PLACEMENT_3D ( 'NONE', #13381, #4176, #4090 ) ;
#5062=EDGE_CURVE ( 'NONE', #13370, #15071, #10010, .T. ) ;
#5063=EDGE_LOOP ( 'NONE', ( #6939, #10922, #14969, #10933 ) ) ;
#5064=ORIENTED_EDGE ( 'NONE', *, *, #2799, .T. ) ;
#5082=AXIS2_PLACEMENT_3D ( 'NONE', #7144, #4626, #2298 ) ;
#5111=CIRCLE ( 'NONE', #5849, 4.000000000000000000 ) ;
#5115=ORIENTED_EDGE ( 'NONE', *, *, #3525, .F. ) ;
#5120=PLANE ( 'NONE',  #12335 ) ;
#5121=EDGE_CURVE ( 'NONE', #241, #4343, #1428, .T. ) ;
#5123=VECTOR ( 'NONE', #3273, 1000.000000000000000 ) ;
#5131=SURFACE_STYLE_FILL_AREA ( #13487 ) ;
#5132=DIRECTION ( 'NONE',  ( 1.000000000000000000, 0.000000000000000000, 0.000000000000000000 ) ) ;
#5134=LINE ( 'NONE', #6191, #2892 ) ;
#5136=EDGE_CURVE ( 'NONE', #6170, #7177, #4818, .T. ) ;
#5138=DIRECTION ( 'NONE',  ( -0.2314933715733012709, 0.9728364810787193395, 0.000000000000000000 ) ) ;
#5150=DIRECTION ( 'NONE',  ( 0.000000000000000000, 0.000000000000000000, 1.000000000000000000 ) ) ;
#5154=FACE_OUTER_BOUND ( 'NONE', #2589, .T. ) ;
#5160=DIRECTION ( 'NONE',  ( 1.000000000000000000, 0.000000000000000000, 0.000000000000000000 ) ) ;
#5170=ORIENTED_EDGE ( 'NONE', *, *, #9384, .T. ) ;
#5172=EDGE_CURVE ( 'NONE', #4384, #7177, #3016, .T. ) ;
#5173=CARTESIAN_POINT ( 'NONE',  ( 0.000000000000000000, 0.000000000000000000, 4.000000000000000000 ) ) ;
#5183=ORIENTED_EDGE ( 'NONE', *, *, #7853, .F. ) ;
#5184=ORIENTED_EDGE ( 'NONE', *, *, #9459, .T. ) ;
#5204=FACE_BOUND ( 'NONE', #12231, .T. ) ;
#5206=( LENGTH_UNIT ( ) NAMED_UNIT ( * ) SI_UNIT ( .MILLI., .METRE. ) );
#5209=EDGE_LOOP ( 'NONE', ( #1708, #700, #14680, #8165 ) ) ;
#5217=CYLINDRICAL_SURFACE ( 'NONE', #12206, 1.999999999999998668 ) ;
#5228=AXIS2_PLACEMENT_3D ( 'NONE', #1506, #12097, #3894 ) ;
#5234=VERTEX_POINT ( 'NONE', #7932 ) ;
#5235=VERTEX_POINT ( 'NONE', #2173 ) ;
#5246=CARTESIAN_POINT ( 'NONE',  ( 72.68384697807672978, 11.35494834827056110, -2.000000000000000888 ) ) ;
#5273=AXIS2_PLACEMENT_3D ( 'NONE', #12039, #1521, #1601 ) ;
#5274=ORIENTED_EDGE ( 'NONE', *, *, #3525, .T. ) ;
#5279=( NAMED_UNIT ( * ) PLANE_ANGLE_UNIT ( ) SI_UNIT ( $, .RADIAN. ) );
#5303=AXIS2_PLACEMENT_3D ( 'NONE', #10258, #14958, #2186 ) ;
#5324=ORIENTED_EDGE ( 'NONE', *, *, #2107, .T. ) ;
#5341=CARTESIAN_POINT ( 'NONE',  ( 13.78117670802322259, -24.07785181381190753, -2.000000000000000000 ) ) ;
#5356=CARTESIAN_POINT ( 'NONE',  ( 18.87754531448929995, -24.24225080111726527, 5.000000000000000000 ) ) ;
#5359=ORIENTED_EDGE ( 'NONE', *, *, #2204, .F. ) ;
#5403=DIRECTION ( 'NONE',  ( 1.000000000000000000, 0.000000000000000000, 0.000000000000000000 ) ) ;
#5416=DIRECTION ( 'NONE',  ( 0.9863939238321436376, 0.1643989873053573192, 0.000000000000000000 ) ) ;
#5431=FACE_OUTER_BOUND ( 'NONE', #5209, .T. ) ;
#5432=ORIENTED_EDGE ( 'NONE', *, *, #9553, .T. ) ;
#5442=ADVANCED_FACE ( 'NONE', ( #1240 ), #4942, .T. ) ;
#5444=ORIENTED_EDGE ( 'NONE', *, *, #3302, .T. ) ;
#5447=CARTESIAN_POINT ( 'NONE',  ( 56.98919079003883326, 3.953582723775848962, -2.000000000000000888 ) ) ;
#5453=ORIENTED_EDGE ( 'NONE', *, *, #2799, .F. ) ;
#5477=EDGE_LOOP ( 'NONE', ( #13122, #4208, #7512, #5801 ) ) ;
#5479=VECTOR ( 'NONE', #5494, 1000.000000000000000 ) ;
#5486=APPLICATION_CONTEXT ( 'automotive_design' ) ;
#5488=EDGE_CURVE ( 'NONE', #10393, #14849, #14479, .T. ) ;
#5494=DIRECTION ( 'NONE',  ( -0.000000000000000000, -0.000000000000000000, 1.000000000000000000 ) ) ;
#5496=DIRECTION ( 'NONE',  ( -0.000000000000000000, -0.000000000000000000, -1.000000000000000000 ) ) ;
#5498=VERTEX_POINT ( 'NONE', #1700 ) ;
#5512=ORIENTED_EDGE ( 'NONE', *, *, #11813, .F. ) ;
#5529=CARTESIAN_POINT ( 'NONE',  ( 18.21994936526786901, -20.29667510578869027, 4.000000000000001776 ) ) ;
#5544=EDGE_CURVE ( 'NONE', #2656, #8622, #8756, .T. ) ;
#5575=EDGE_LOOP ( 'NONE', ( #3433, #6074 ) ) ;
#5578=DIRECTION ( 'NONE',  ( -0.9863939238321437486, -0.1643989873053574857, 0.000000000000000000 ) ) ;
#5587=ORIENTED_EDGE ( 'NONE', *, *, #9619, .T. ) ;
#5604=VERTEX_POINT ( 'NONE', #6533 ) ;
#5609=CARTESIAN_POINT ( 'NONE',  ( 88.84370878116858705, 10.64188714589527684, 7.000000000000000000 ) ) ;
#5619=CARTESIAN_POINT ( 'NONE',  ( 64.00448238961524794, 36.25062540154047497, -2.000000000000000000 ) ) ;
#5638=CARTESIAN_POINT ( 'NONE',  ( 93.63799900313688340, -2.337932895214617890, -2.000000000000000888 ) ) ;
#5641=VECTOR ( 'NONE', #2503, 1000.000000000000000 ) ;
#5657=AXIS2_PLACEMENT_3D ( 'NONE', #10678, #2227, #1147 ) ;
#5663=ORIENTED_EDGE ( 'NONE', *, *, #10042, .F. ) ;
#5666=VERTEX_POINT ( 'NONE', #3300 ) ;
#5717=DIRECTION ( 'NONE',  ( 0.000000000000000000, 0.000000000000000000, 1.000000000000000000 ) ) ;
#5718=CARTESIAN_POINT ( 'NONE',  ( 64.00448238961524794, 36.25062540154047497, 5.000000000000000888 ) ) ;
#5719=ORIENTED_EDGE ( 'NONE', *, *, #4293, .T. ) ;
#5723=ADVANCED_FACE ( 'NONE', ( #4696 ), #10749, .T. ) ;
#5725=EDGE_LOOP ( 'NONE', ( #3568, #5432, #1320, #3164, #11754, #10810, #6498, #10309 ) ) ;
#5730=DIRECTION ( 'NONE',  ( 1.000000000000000000, 0.000000000000000000, 0.000000000000000000 ) ) ;
#5738=FACE_OUTER_BOUND ( 'NONE', #5063, .T. ) ;
#5740=DIRECTION ( 'NONE',  ( 0.1643989873053574580, -0.9863939238321436376, 0.000000000000000000 ) ) ;
#5742=CARTESIAN_POINT ( 'NONE',  ( 98.48580539929344013, 0.9022481406819604643, 4.000000000000000000 ) ) ;
#5779=AXIS2_PLACEMENT_3D ( 'NONE', #14890, #11414, #3352 ) ;
#5787=ORIENTED_EDGE ( 'NONE', *, *, #10614, .F. ) ;
#5795=VERTEX_POINT ( 'NONE', #6982 ) ;
#5801=ORIENTED_EDGE ( 'NONE', *, *, #9063, .F. ) ;
#5831=CARTESIAN_POINT ( 'NONE',  ( 60.23740434540291488, 32.40236306526279719, 7.000000000000000000 ) ) ;
#5833=VECTOR ( 'NONE', #15195, 1000.000000000000000 ) ;
#5841=EDGE_CURVE ( 'NONE', #8240, #13379, #4925, .T. ) ;
#5849=AXIS2_PLACEMENT_3D ( 'NONE', #11938, #14028, #4899 ) ;
#5856=ORIENTED_EDGE ( 'NONE', *, *, #1020, .F. ) ;
#5866=CIRCLE ( 'NONE', #14456, 2.999999999999988898 ) ;
#5886=ORIENTED_EDGE ( 'NONE', *, *, #4133, .T. ) ;
#5895=CARTESIAN_POINT ( 'NONE',  ( 91.12964445316929130, 15.08873975234342701, -2.000000000000000888 ) ) ;
#5898=CARTESIAN_POINT ( 'NONE',  ( 13.78117670802322259, -24.07785181381190753, -2.000000000000000000 ) ) ;
#5901=FACE_OUTER_BOUND ( 'NONE', #2871, .T. ) ;
#5903=AXIS2_PLACEMENT_3D ( 'NONE', #582, #3981, #356 ) ;
#5907=ADVANCED_FACE ( 'NONE', ( #7446 ), #9826, .F. ) ;
#5909=ORIENTED_EDGE ( 'NONE', *, *, #6665, .F. ) ;
#5912=LINE ( 'NONE', #3444, #1900 ) ;
#5922=FACE_OUTER_BOUND ( 'NONE', #10474, .T. ) ;
#5924=EDGE_CURVE ( 'NONE', #3172, #3460, #226, .T. ) ;
#5931=ADVANCED_FACE ( 'NONE', ( #1752 ), #6434, .T. ) ;
#5936=LINE ( 'NONE', #3693, #1886 ) ;
#5937=ORIENTED_EDGE ( 'NONE', *, *, #5841, .T. ) ;
#5938=LINE ( 'NONE', #8233, #2584 ) ;
#5943=ORIENTED_EDGE ( 'NONE', *, *, #2401, .T. ) ;
#5948=DIRECTION ( 'NONE',  ( 1.000000000000000000, 0.000000000000000000, 0.000000000000000000 ) ) ;
#5956=CARTESIAN_POINT ( 'NONE',  ( 58.14665764790533586, -0.9105996816177489572, -2.000000000000000888 ) ) ;
#5958=LINE ( 'NONE', #8403, #2649 ) ;
#5961=LINE ( 'NONE', #8186, #14738 ) ;
#5969=ADVANCED_FACE ( 'NONE', ( #7291 ), #7900, .F. ) ;
#5970=ORIENTED_EDGE ( 'NONE', *, *, #13137, .F. ) ;
#5973=CYLINDRICAL_SURFACE ( 'NONE', #13699, 3.000000000000002665 ) ;
#5986=CARTESIAN_POINT ( 'NONE',  ( 19.20634328910001543, -26.21503864878155099, 4.000000000000000000 ) ) ;
#5995=LINE ( 'NONE', #8220, #1440 ) ;
#5997=CARTESIAN_POINT ( 'NONE',  ( -9.999999999999998224, -1.390791565672605534, 7.000000000000000000 ) ) ;
#6000=VECTOR ( 'NONE', #10631, 1000.000000000000000 ) ;
#6003=ORIENTED_EDGE ( 'NONE', *, *, #8807, .T. ) ;
#6016=CARTESIAN_POINT ( 'NONE',  ( 18.21994936526786901, -20.29667510578869027, 7.000000000000000000 ) ) ;
#6032=DIRECTION ( 'NONE',  ( -0.000000000000000000, -0.000000000000000000, 1.000000000000000000 ) ) ;
#6033=DIRECTION ( 'NONE',  ( -0.9148936170212769170, -0.4036950204470262649, 0.000000000000000000 ) ) ;
#6053=AXIS2_PLACEMENT_3D ( 'NONE', #5356, #8701, #13479 ) ;
#6060=DIRECTION ( 'NONE',  ( 1.000000000000000000, 0.000000000000000000, 0.000000000000000000 ) ) ;
#6074=ORIENTED_EDGE ( 'NONE', *, *, #8709, .T. ) ;
#6083=EDGE_LOOP ( 'NONE', ( #6325, #3222, #2674, #6951 ) ) ;
#6087=EDGE_CURVE ( 'NONE', #14849, #4961, #5961, .T. ) ;
#6089=VECTOR ( 'NONE', #3761, 1000.000000000000114 ) ;
#6098=ORIENTED_EDGE ( 'NONE', *, *, #4941, .T. ) ;
#6105=VECTOR ( 'NONE', #8084, 1000.000000000000000 ) ;
#6113=ORIENTED_EDGE ( 'NONE', *, *, #12202, .T. ) ;
#6144=ADVANCED_FACE ( 'NONE', ( #1268, #8263 ), #10645, .T. ) ;
#6147=ORIENTED_EDGE ( 'NONE', *, *, #10614, .T. ) ;
#6149=EDGE_LOOP ( 'NONE', ( #10437, #2631, #12058, #8857 ) ) ;
#6152=FACE_OUTER_BOUND ( 'NONE', #12485, .T. ) ;
#6153=FACE_OUTER_BOUND ( 'NONE', #11585, .T. ) ;
#6163=CARTESIAN_POINT ( 'NONE',  ( -9.999999999999992895, -25.00000000000000000, 7.000000000000000000 ) ) ;
#6170=VERTEX_POINT ( 'NONE', #5898 ) ;
#6174=DIRECTION ( 'NONE',  ( 0.000000000000000000, 0.000000000000000000, 1.000000000000000000 ) ) ;
#6187=DIRECTION ( 'NONE',  ( 0.000000000000000000, 0.000000000000000000, 1.000000000000000000 ) ) ;
#6190=ADVANCED_FACE ( 'NONE', ( #13178 ), #8571, .F. ) ;
#6191=CARTESIAN_POINT ( 'NONE',  ( 18.71314632718394222, -23.25585687728512241, -2.000000000000000000 ) ) ;
#6193=DIRECTION ( 'NONE',  ( 0.9148936170212768060, 0.4036950204470267645, -0.000000000000000000 ) ) ;
#6256=EDGE_CURVE ( 'NONE', #2817, #15071, #5134, .T. ) ;
#6268=CYLINDRICAL_SURFACE ( 'NONE', #13049, 4.000000000000000000 ) ;
#6298=DIRECTION ( 'NONE',  ( 0.000000000000000000, 0.000000000000000000, 1.000000000000000000 ) ) ;
#6314=VECTOR ( 'NONE', #3041, 1000.000000000000114 ) ;
#6325=ORIENTED_EDGE ( 'NONE', *, *, #4509, .T. ) ;
#6341=CARTESIAN_POINT ( 'NONE',  ( 75.68384697807671557, 11.35494834827056110, 4.000000000000000000 ) ) ;
#6348=CARTESIAN_POINT ( 'NONE',  ( 4.000000000000000000, 4.898587196589412829E-16, 4.500000000000000888 ) ) ;
#6353=ORIENTED_EDGE ( 'NONE', *, *, #10308, .F. ) ;
#6356=DIRECTION ( 'NONE',  ( 1.000000000000000000, 0.000000000000000000, 0.000000000000000000 ) ) ;
#6371=CARTESIAN_POINT ( 'NONE',  ( 70.16198417812034904, 9.730076655429538590, -2.000000000000000888 ) ) ;
#6376=ORIENTED_EDGE ( 'NONE', *, *, #2998, .F. ) ;
#6385=CARTESIAN_POINT ( 'NONE',  ( 10.00000000000000178, -1.390791565672601315, 7.000000000000006217 ) ) ;
#6405=DIRECTION ( 'NONE',  ( 1.000000000000000000, 0.000000000000000000, 0.000000000000000000 ) ) ;
#6416=ADVANCED_FACE ( 'NONE', ( #6653 ), #11397, .F. ) ;
#6434=PLANE ( 'NONE',  #5903 ) ;
#6437=CARTESIAN_POINT ( 'NONE',  ( 80.00000000000000000, 0.000000000000000000, 4.000000000000003553 ) ) ;
#6441=DIRECTION ( 'NONE',  ( -0.000000000000000000, -0.000000000000000000, -1.000000000000000000 ) ) ;
#6447=ORIENTED_EDGE ( 'NONE', *, *, #12767, .T. ) ;
#6448=( NAMED_UNIT ( * ) SI_UNIT ( $, .STERADIAN. ) SOLID_ANGLE_UNIT ( ) );
#6458=ORIENTED_EDGE ( 'NONE', *, *, #12667, .T. ) ;
#6462=EDGE_LOOP ( 'NONE', ( #11520, #11943, #5359, #7331 ) ) ;
#6473=CARTESIAN_POINT ( 'NONE',  ( 64.00448238961524794, 36.25062540154047497, -8.169391093593850073 ) ) ;
#6483=VECTOR ( 'NONE', #14522, 1000.000000000000000 ) ;
#6498=ORIENTED_EDGE ( 'NONE', *, *, #7988, .T. ) ;
#6502=CIRCLE ( 'NONE', #3552, 9.999999999999994671 ) ;
#6504=ORIENTED_EDGE ( 'NONE', *, *, #6256, .F. ) ;
#6533=CARTESIAN_POINT ( 'NONE',  ( 55.83172393217232354, 8.817765129169439220, 7.000000000000000000 ) ) ;
#6537=DIRECTION ( 'NONE',  ( -0.000000000000000000, -0.000000000000000000, -1.000000000000000000 ) ) ;
#6549=AXIS2_PLACEMENT_3D ( 'NONE', #10094, #4260, #8936 ) ;
#6552=DIRECTION ( 'NONE',  ( 0.1643989873053580408, -0.9863939238321435266, -0.000000000000000000 ) ) ;
#6567=CIRCLE ( 'NONE', #12689, 2.999999999999988898 ) ;
#6568=ORIENTED_EDGE ( 'NONE', *, *, #5544, .F. ) ;
#6569=ORIENTED_EDGE ( 'NONE', *, *, #11440, .T. ) ;
#6581=DIRECTION ( 'NONE',  ( 0.9863939238321437486, 0.1643989873053574857, -0.000000000000000000 ) ) ;
#6593=DIRECTION ( 'NONE',  ( 1.000000000000000000, 0.000000000000000000, 0.000000000000000000 ) ) ;
#6594=AXIS2_PLACEMENT_3D ( 'NONE', #3030, #10382, #7718 ) ;
#6600=LINE ( 'NONE', #7337, #6725 ) ;
#6626=VERTEX_POINT ( 'NONE', #10786 ) ;
#6630=AXIS2_PLACEMENT_3D ( 'NONE', #6385, #12134, #9688 ) ;
#6641=CARTESIAN_POINT ( 'NONE',  ( 62.65957446808508280, 26.91300136313512681, 7.000000000000000000 ) ) ;
#6647=EDGE_LOOP ( 'NONE', ( #8478, #8489, #12927, #11948 ) ) ;
#6653=FACE_OUTER_BOUND ( 'NONE', #7730, .T. ) ;
#6665=EDGE_CURVE ( 'NONE', #13379, #8240, #13194, .T. ) ;
#6672=EDGE_LOOP ( 'NONE', ( #7944, #1735, #9983, #10653 ) ) ;
#6682=CARTESIAN_POINT ( 'NONE',  ( -9.999999999999998224, 0.000000000000000000, 7.000000000000000000 ) ) ;
#6683=VERTEX_POINT ( 'NONE', #8323 ) ;
#6687=VECTOR ( 'NONE', #3660, 1000.000000000000000 ) ;
#6698=VERTEX_POINT ( 'NONE', #10854 ) ;
#6709=LINE ( 'NONE', #4336, #872 ) ;
#6715=DIRECTION ( 'NONE',  ( 1.000000000000000000, 0.000000000000000000, 0.000000000000000000 ) ) ;
#6719=ORIENTED_EDGE ( 'NONE', *, *, #3928, .T. ) ;
#6725=VECTOR ( 'NONE', #3634, 1000.000000000000114 ) ;
#6727=ORIENTED_EDGE ( 'NONE', *, *, #8757, .T. ) ;
#6743=DIRECTION ( 'NONE',  ( -0.5416238976136773520, 0.8406209333187989463, 0.000000000000000000 ) ) ;
#6761=AXIS2_PLACEMENT_3D ( 'NONE', #11546, #4490, #12772 ) ;
#6763=DIRECTION ( 'NONE',  ( 0.1643989873053574580, -0.9863939238321436376, 0.000000000000000000 ) ) ;
#6765=EDGE_CURVE ( 'NONE', #10729, #8622, #7706, .T. ) ;
#6767=LINE ( 'NONE', #2006, #8245 ) ;
#6781=ORIENTED_EDGE ( 'NONE', *, *, #14695, .F. ) ;
#6784=CARTESIAN_POINT ( 'NONE',  ( 83.50748565343083385, 13.38500995229612478, -2.000000000000000888 ) ) ;
#6788=DIRECTION ( 'NONE',  ( -0.9148936170212765839, -0.4036950204470272086, 0.000000000000000000 ) ) ;
#6790=EDGE_LOOP ( 'NONE', ( #2493, #12046 ) ) ;
#6802=ORIENTED_EDGE ( 'NONE', *, *, #9963, .T. ) ;
#6820=DIRECTION ( 'NONE',  ( -0.000000000000000000, -0.000000000000000000, 1.000000000000000000 ) ) ;
#6823=EDGE_CURVE ( 'NONE', #2548, #14792, #12474, .T. ) ;
#6827=VERTEX_POINT ( 'NONE', #2019 ) ;
#6828=VECTOR ( 'NONE', #4063, 1000.000000000000227 ) ;
#6832=CARTESIAN_POINT ( 'NONE',  ( 72.49759028996471955, 17.18292470770558822, 7.000000000000000000 ) ) ;
#6833=ORIENTED_EDGE ( 'NONE', *, *, #4957, .T. ) ;
#6836=CARTESIAN_POINT ( 'NONE',  ( 55.83172393217232354, 8.817765129169439220, -2.000000000000000888 ) ) ;
#6858=VECTOR ( 'NONE', #1342, 1000.000000000000000 ) ;
#6868=CYLINDRICAL_SURFACE ( 'NONE', #11909, 20.00000000000000000 ) ;
#6873=AXIS2_PLACEMENT_3D ( 'NONE', #1679, #8734, #9746 ) ;
#6881=CARTESIAN_POINT ( 'NONE',  ( 60.23740434540291488, 32.40236306526279009, 7.000000000000000000 ) ) ;
#6926=DIRECTION ( 'NONE',  ( 0.9728364810787193395, 0.2314933715733012709, -0.000000000000000000 ) ) ;
#6935=AXIS2_PLACEMENT_3D ( 'NONE', #14576, #4044, #12261 ) ;
#6939=ORIENTED_EDGE ( 'NONE', *, *, #915, .F. ) ;
#6941=DIRECTION ( 'NONE',  ( 1.000000000000000000, 0.000000000000000000, 0.000000000000000000 ) ) ;
#6951=ORIENTED_EDGE ( 'NONE', *, *, #12420, .F. ) ;
#6960=LINE ( 'NONE', #5895, #9020 ) ;
#6964=ORIENTED_EDGE ( 'NONE', *, *, #11239, .T. ) ;
#6974=EDGE_LOOP ( 'NONE', ( #12589, #6003, #13740, #4168 ) ) ;
#6975=AXIS2_PLACEMENT_3D ( 'NONE', #13070, #11924, #1412 ) ;
#6982=CARTESIAN_POINT ( 'NONE',  ( 91.12964445316927709, 15.08873975234342701, 4.000000000000000000 ) ) ;
#6984=AXIS2_PLACEMENT_3D ( 'NONE', #3762, #138, #9767 ) ;
#6990=LINE ( 'NONE', #3523, #12862 ) ;
#6998=CARTESIAN_POINT ( 'NONE',  ( 85.79342132543153809, 17.83186255874426962, -2.000000000000000888 ) ) ;
#7004=DIRECTION ( 'NONE',  ( -0.000000000000000000, -0.000000000000000000, 1.000000000000000000 ) ) ;
#7005=AXIS2_PLACEMENT_3D ( 'NONE', #13856, #5578, #873 ) ;
#7010=CARTESIAN_POINT ( 'NONE',  ( 75.20570977803312473, 12.97982004111159959, -2.000000000000000888 ) ) ;
#7015=EDGE_CURVE ( 'NONE', #5666, #12669, #7567, .T. ) ;
#7021=AXIS2_PLACEMENT_3D ( 'NONE', #10973, #4064, #9666 ) ;
#7032=LINE ( 'NONE', #3570, #9048 ) ;
#7042=DIRECTION ( 'NONE',  ( 0.000000000000000000, 0.000000000000000000, 1.000000000000000000 ) ) ;
#7068=DIRECTION ( 'NONE',  ( 0.9148936170212765839, 0.4036950204470272086, -0.000000000000000000 ) ) ;
#7070=ORIENTED_EDGE ( 'NONE', *, *, #11956, .T. ) ;
#7081=DIRECTION ( 'NONE',  ( 0.4036950204470249881, -0.9148936170212775831, 0.000000000000000000 ) ) ;
#7094=ORIENTED_EDGE ( 'NONE', *, *, #9384, .F. ) ;
#7107=DIRECTION ( 'NONE',  ( -0.000000000000000000, -0.000000000000000000, 1.000000000000000000 ) ) ;
#7112=LINE ( 'NONE', #5956, #13189 ) ;
#7123=AXIS2_PLACEMENT_3D ( 'NONE', #7358, #7503, #4039 ) ;
#7125=EDGE_CURVE ( 'NONE', #1757, #6626, #10021, .T. ) ;
#7126=VERTEX_POINT ( 'NONE', #13349 ) ;
#7128=EDGE_CURVE ( 'NONE', #14060, #4311, #10757, .T. ) ;
#7137=CARTESIAN_POINT ( 'NONE',  ( 98.33955663538051795, 3.898681236723621879, 7.000000000000000000 ) ) ;
#7144=CARTESIAN_POINT ( 'NONE',  ( 98.48580539929344013, 0.9022481406819604643, -2.000000000000000888 ) ) ;
#7147=VERTEX_POINT ( 'NONE', #9892 ) ;
#7150=ORIENTED_EDGE ( 'NONE', *, *, #11812, .F. ) ;
#7154=CARTESIAN_POINT ( 'NONE',  ( 85.79342132543153809, 17.83186255874426962, 7.000000000000000000 ) ) ;
#7156=EDGE_CURVE ( 'NONE', #14360, #10918, #9751, .T. ) ;
#7161=VECTOR ( 'NONE', #14753, 1000.000000000000114 ) ;
#7177=VERTEX_POINT ( 'NONE', #10280 ) ;
#7178=LINE ( 'NONE', #6881, #2282 ) ;
#7179=ADVANCED_FACE ( 'NONE', ( #9202 ), #13659, .F. ) ;
#7181=ORIENTED_EDGE ( 'NONE', *, *, #10529, .T. ) ;
#7183=ORIENTED_EDGE ( 'NONE', *, *, #11956, .F. ) ;
#7192=ORIENTED_EDGE ( 'NONE', *, *, #7835, .F. ) ;
#7202=DIRECTION ( 'NONE',  ( -0.000000000000000000, -0.000000000000000000, 1.000000000000000000 ) ) ;
#7218=ORIENTED_EDGE ( 'NONE', *, *, #12503, .T. ) ;
#7248=VERTEX_POINT ( 'NONE', #975 ) ;
#7253=DIRECTION ( 'NONE',  ( 0.1643989873053574580, -0.9863939238321436376, 0.000000000000000000 ) ) ;
#7254=DIRECTION ( 'NONE',  ( 1.000000000000000000, 0.000000000000000000, 0.000000000000000000 ) ) ;
#7256=CARTESIAN_POINT ( 'NONE',  ( 61.98919079003883326, 3.953582723775848962, -2.000000000000000888 ) ) ;
#7258=VERTEX_POINT ( 'NONE', #2052 ) ;
#7291=FACE_OUTER_BOUND ( 'NONE', #128, .T. ) ;
#7303=CIRCLE ( 'NONE', #14429, 4.000000000000003553 ) ;
#7315=DIRECTION ( 'NONE',  ( 1.000000000000000000, 0.000000000000000000, 0.000000000000000000 ) ) ;
#7318=EDGE_LOOP ( 'NONE', ( #5064, #5170 ) ) ;
#7328=LINE ( 'NONE', #6163, #9947 ) ;
#7331=ORIENTED_EDGE ( 'NONE', *, *, #8973, .F. ) ;
#7337=CARTESIAN_POINT ( 'NONE',  ( 33.82574562093736859, -6.697933970950280091, 7.000000000000000000 ) ) ;
#7338=DIRECTION ( 'NONE',  ( 0.000000000000000000, 0.000000000000000000, 1.000000000000000000 ) ) ;
#7353=CARTESIAN_POINT ( 'NONE',  ( 0.000000000000000000, 0.000000000000000000, 0.000000000000000000 ) ) ;
#7358=CARTESIAN_POINT ( 'NONE',  ( 88.46153288930041469, 16.46030115554384565, -2.000000000000000888 ) ) ;
#7360=DIRECTION ( 'NONE',  ( -0.9728364810787193395, -0.2314933715733012709, 0.000000000000000000 ) ) ;
#7361=CARTESIAN_POINT ( 'NONE',  ( 32.66827876307085887, -1.833751565556681173, 7.000000000000000000 ) ) ;
#7362=DIRECTION ( 'NONE',  ( 1.000000000000000000, 0.000000000000000000, 0.000000000000000000 ) ) ;
#7367=ORIENTED_EDGE ( 'NONE', *, *, #2860, .F. ) ;
#7375=ORIENTED_EDGE ( 'NONE', *, *, #6823, .T. ) ;
#7379=ORIENTED_EDGE ( 'NONE', *, *, #15025, .T. ) ;
#7387=LINE ( 'NONE', #7455, #12413 ) ;
#7389=ORIENTED_EDGE ( 'NONE', *, *, #8095, .F. ) ;
#7393=EDGE_CURVE ( 'NONE', #5234, #7126, #13963, .T. ) ;
#7398=CARTESIAN_POINT ( 'NONE',  ( -4.000000000000000000, 0.000000000000000000, 4.000000000000000000 ) ) ;
#7411=ADVANCED_FACE ( 'NONE', ( #8573 ), #1578, .F. ) ;
#7412=ADVANCED_FACE ( 'NONE', ( #3728 ), #1505, .T. ) ;
#7429=ORIENTED_EDGE ( 'NONE', *, *, #4240, .F. ) ;
#7435=EDGE_LOOP ( 'NONE', ( #7644, #7998, #2760, #8050, #3040 ) ) ;
#7441=CARTESIAN_POINT ( 'NONE',  ( 83.50748565343083385, 13.38500995229612478, 7.000000000000000000 ) ) ;
#7446=FACE_OUTER_BOUND ( 'NONE', #5725, .T. ) ;
#7455=CARTESIAN_POINT ( 'NONE',  ( -9.999999999999998224, 0.000000000000000000, -130.1575142076926852 ) ) ;
#7457=EDGE_LOOP ( 'NONE', ( #10270, #9082, #8879, #7735 ) ) ;
#7460=DIRECTION ( 'NONE',  ( 1.000000000000000000, 0.000000000000000000, 0.000000000000000000 ) ) ;
#7467=ORIENTED_EDGE ( 'NONE', *, *, #12634, .F. ) ;
#7470=VERTEX_POINT ( 'NONE', #9645 ) ;
#7477=UNCERTAINTY_MEASURE_WITH_UNIT (LENGTH_MEASURE( 1.000000000000000082E-05 ), #3886, 'distance_accuracy_value', 'NONE');
#7482=VECTOR ( 'NONE', #11829, 1000.000000000000227 ) ;
#7489=DIRECTION ( 'NONE',  ( 0.9148936170212769170, 0.4036950204470268200, -0.000000000000000000 ) ) ;
#7503=DIRECTION ( 'NONE',  ( -0.000000000000000000, -0.000000000000000000, 1.000000000000000000 ) ) ;
#7512=ORIENTED_EDGE ( 'NONE', *, *, #2396, .T. ) ;
#7515=DIRECTION ( 'NONE',  ( 0.000000000000000000, 0.000000000000000000, 1.000000000000000000 ) ) ;
#7516=CARTESIAN_POINT ( 'NONE',  ( 0.000000000000000000, 0.000000000000000000, 4.500000000000000888 ) ) ;
#7517=ADVANCED_FACE ( 'NONE', ( #9727 ), #11032, .T. ) ;
#7521=PLANE ( 'NONE',  #13308 ) ;
#7532=VECTOR ( 'NONE', #8128, 1000.000000000000114 ) ;
#7539=DIRECTION ( 'NONE',  ( 0.000000000000000000, 0.000000000000000000, 1.000000000000000000 ) ) ;
#7556=CARTESIAN_POINT ( 'NONE',  ( 0.3363705501000965326, -6.891763197764913862, 4.000000000000000000 ) ) ;
#7565=ADVANCED_FACE ( 'NONE', ( #13181 ), #2667, .F. ) ;
#7567=CIRCLE ( 'NONE', #11957, 2.000000000000003109 ) ;
#7580=AXIS2_PLACEMENT_3D ( 'NONE', #100, #4823, #4907 ) ;
#7597=PRODUCT_CONTEXT ( 'NONE', #1833, 'mechanical' ) ;
#7598=DIRECTION ( 'NONE',  ( 0.000000000000000000, 0.000000000000000000, 1.000000000000000000 ) ) ;
#7602=DIRECTION ( 'NONE',  ( -0.4036950204470279302, 0.9148936170212763619, 0.000000000000000000 ) ) ;
#7620=ORIENTED_EDGE ( 'NONE', *, *, #3365, .T. ) ;
#7622=CARTESIAN_POINT ( 'NONE',  ( 88.46153288930041469, 16.46030115554384565, 4.000000000000000000 ) ) ;
#7633=ORIENTED_EDGE ( 'NONE', *, *, #2998, .T. ) ;
#7644=ORIENTED_EDGE ( 'NONE', *, *, #8412, .T. ) ;
#7680=DIRECTION ( 'NONE',  ( 1.000000000000000000, 0.000000000000000000, 0.000000000000000000 ) ) ;
#7681=VECTOR ( 'NONE', #12547, 1000.000000000000000 ) ;
#7702=CARTESIAN_POINT ( 'NONE',  ( 18.71314632718394222, -23.25585687728512241, 2.000000000000000000 ) ) ;
#7706=LINE ( 'NONE', #6473, #4127 ) ;
#7711=CIRCLE ( 'NONE', #3776, 2.999999999999975131 ) ;
#7712=ORIENTED_EDGE ( 'NONE', *, *, #2776, .T. ) ;
#7717=ORIENTED_EDGE ( 'NONE', *, *, #14272, .F. ) ;
#7718=DIRECTION ( 'NONE',  ( 1.000000000000000000, 0.000000000000000000, 0.000000000000000000 ) ) ;
#7724=VECTOR ( 'NONE', #10896, 1000.000000000000000 ) ;
#7730=EDGE_LOOP ( 'NONE', ( #12067, #14757, #3290, #3883 ) ) ;
#7735=ORIENTED_EDGE ( 'NONE', *, *, #12147, .F. ) ;
#7757=CARTESIAN_POINT ( 'NONE',  ( 65.21556745095632834, 33.50594455047664866, -2.000000000000000000 ) ) ;
#7769=DIRECTION ( 'NONE',  ( -0.000000000000000000, -0.000000000000000000, 1.000000000000000000 ) ) ;
#7772=EDGE_CURVE ( 'NONE', #8240, #3993, #12708, .T. ) ;
#7781=STYLED_ITEM('',(#15265),#13393);
#7796=DIRECTION ( 'NONE',  ( -0.000000000000000000, -0.000000000000000000, 1.000000000000000000 ) ) ;
#7806=AXIS2_PLACEMENT_3D ( 'NONE', #5638, #10461, #3465 ) ;
#7811=CIRCLE ( 'NONE', #12468, 4.000000000000000000 ) ;
#7821=CARTESIAN_POINT ( 'NONE',  ( 101.6227766016837819, 5.204170427930421283E-15, 7.000000000000006217 ) ) ;
#7829=CARTESIAN_POINT ( 'NONE',  ( 98.63205416320636232, -2.094184955359725375, -2.000000000000000888 ) ) ;
#7835=EDGE_CURVE ( 'NONE', #10776, #1519, #10488, .T. ) ;
#7852=DIRECTION ( 'NONE',  ( -0.000000000000000000, -0.000000000000000000, 1.000000000000000000 ) ) ;
#7853=EDGE_CURVE ( 'NONE', #3507, #3292, #2723, .T. ) ;
#7862=LINE ( 'NONE', #12538, #13376 ) ;
#7876=VERTEX_POINT ( 'NONE', #4956 ) ;
#7877=EDGE_CURVE ( 'NONE', #11474, #8331, #11013, .T. ) ;
#7878=CYLINDRICAL_SURFACE ( 'NONE', #9219, 4.999999999999997335 ) ;
#7895=EDGE_CURVE ( 'NONE', #7177, #1861, #478, .T. ) ;
#7897=CARTESIAN_POINT ( 'NONE',  ( 55.83172393217232354, 8.817765129169439220, 4.000000000000000000 ) ) ;
#7900=CYLINDRICAL_SURFACE ( 'NONE', #11295, 4.999999999999997335 ) ;
#7920=ORIENTED_EDGE ( 'NONE', *, *, #1459, .T. ) ;
#7927=ORIENTED_EDGE ( 'NONE', *, *, #14839, .F. ) ;
#7932=CARTESIAN_POINT ( 'NONE',  ( 70.16198417812034904, 9.730076655429538590, 7.000000000000000000 ) ) ;
#7944=ORIENTED_EDGE ( 'NONE', *, *, #4665, .F. ) ;
#7962=VECTOR ( 'NONE', #611, 1000.000000000000000 ) ;
#7966=EDGE_LOOP ( 'NONE', ( #2080, #12975, #4369, #4070 ) ) ;
#7968=CARTESIAN_POINT ( 'NONE',  ( 98.33955663538051795, 3.898681236723621879, 4.000000000000000000 ) ) ;
#7988=EDGE_CURVE ( 'NONE', #4008, #8012, #715, .T. ) ;
#7995=CARTESIAN_POINT ( 'NONE',  ( 86.00000000000000000, 0.000000000000000000, 4.500000000000000888 ) ) ;
#7998=ORIENTED_EDGE ( 'NONE', *, *, #8016, .T. ) ;
#8006=ORIENTED_EDGE ( 'NONE', *, *, #2726, .F. ) ;
#8012=VERTEX_POINT ( 'NONE', #13623 ) ;
#8015=DIRECTION ( 'NONE',  ( 1.000000000000000000, 0.000000000000000000, 0.000000000000000000 ) ) ;
#8016=EDGE_CURVE ( 'NONE', #14530, #11965, #330, .T. ) ;
#8028=CARTESIAN_POINT ( 'NONE',  ( 80.00000000000000000, 0.000000000000000000, 4.500000000000003553 ) ) ;
#8050=ORIENTED_EDGE ( 'NONE', *, *, #11352, .T. ) ;
#8055=DIRECTION ( 'NONE',  ( 1.000000000000000000, 0.000000000000000000, 0.000000000000000000 ) ) ;
#8057=LINE ( 'NONE', #13248, #7532 ) ;
#8084=DIRECTION ( 'NONE',  ( -0.000000000000000000, -0.000000000000000000, 1.000000000000000000 ) ) ;
#8095=EDGE_CURVE ( 'NONE', #1504, #6698, #1326, .T. ) ;
#8112=ORIENTED_EDGE ( 'NONE', *, *, #15174, .F. ) ;
#8128=DIRECTION ( 'NONE',  ( -0.9728364810787193395, -0.2314933715733012709, 0.000000000000000000 ) ) ;
#8156=CARTESIAN_POINT ( 'NONE',  ( 0.000000000000000000, 0.000000000000000000, -2.000000000000000000 ) ) ;
#8161=ORIENTED_EDGE ( 'NONE', *, *, #9330, .F. ) ;
#8165=ORIENTED_EDGE ( 'NONE', *, *, #1489, .T. ) ;
#8177=LINE ( 'NONE', #1192, #4097 ) ;
#8186=CARTESIAN_POINT ( 'NONE',  ( 13.28797974610715116, -21.11867004231547540, 7.000000000000000000 ) ) ;
#8198=CIRCLE ( 'NONE', #11874, 4.000000000000003553 ) ;
#8200=FACE_OUTER_BOUND ( 'NONE', #6974, .T. ) ;
#8208=CYLINDRICAL_SURFACE ( 'NONE', #5082, 3.000000000000002665 ) ;
#8220=CARTESIAN_POINT ( 'NONE',  ( -9.999999999999992895, -25.00000000000000000, 4.000000000000003553 ) ) ;
#8221=VECTOR ( 'NONE', #1711, 1000.000000000000227 ) ;
#8223=LINE ( 'NONE', #12898, #6089 ) ;
#8233=CARTESIAN_POINT ( 'NONE',  ( 3.948182771089140175, -23.68909662653485171, 4.000000000000000000 ) ) ;
#8237=CIRCLE ( 'NONE', #10693, 4.999999999999997335 ) ;
#8240=VERTEX_POINT ( 'NONE', #8447 ) ;
#8244=DIRECTION ( 'NONE',  ( -0.000000000000000000, -0.000000000000000000, 1.000000000000000000 ) ) ;
#8245=VECTOR ( 'NONE', #10223, 1000.000000000000000 ) ;
#8260=DIRECTION ( 'NONE',  ( 0.000000000000000000, 0.000000000000000000, 1.000000000000000000 ) ) ;
#8263=FACE_BOUND ( 'NONE', #7318, .T. ) ;
#8314=AXIS2_PLACEMENT_3D ( 'NONE', #5742, #11569, #12864 ) ;
#8322=DIRECTION ( 'NONE',  ( 1.000000000000000000, 0.000000000000000000, 0.000000000000000000 ) ) ;
#8323=CARTESIAN_POINT ( 'NONE',  ( 80.82762530298222714, -9.999999999999994671, 7.000000000000000000 ) ) ;
#8329=CARTESIAN_POINT ( 'NONE',  ( -6.000000000000000888, 7.347880794884120722E-16, 7.000000000000000000 ) ) ;
#8331=VERTEX_POINT ( 'NONE', #14766 ) ;
#8334=FACE_BOUND ( 'NONE', #731, .T. ) ;
#8348=ORIENTED_EDGE ( 'NONE', *, *, #11440, .F. ) ;
#8370=DIRECTION ( 'NONE',  ( -0.1643989873053574580, 0.9863939238321436376, 0.000000000000000000 ) ) ;
#8384=DIRECTION ( 'NONE',  ( -0.1643989873053572359, 0.9863939238321437486, 0.000000000000000000 ) ) ;
#8397=AXIS2_PLACEMENT_3D ( 'NONE', #8656, #9591, #6060 ) ;
#8403=CARTESIAN_POINT ( 'NONE',  ( 88.84370878116858705, 10.64188714589527507, -2.000000000000000888 ) ) ;
#8404=DIRECTION ( 'NONE',  ( 1.000000000000000000, 0.000000000000000000, 0.000000000000000000 ) ) ;
#8410=FACE_OUTER_BOUND ( 'NONE', #5477, .T. ) ;
#8412=EDGE_CURVE ( 'NONE', #10155, #14530, #9717, .T. ) ;
#8415=ORIENTED_EDGE ( 'NONE', *, *, #1758, .T. ) ;
#8420=PLANE ( 'NONE',  #2872 ) ;
#8423=DIRECTION ( 'NONE',  ( 0.000000000000000000, 0.000000000000000000, 1.000000000000000000 ) ) ;
#8441=ORIENTED_EDGE ( 'NONE', *, *, #12147, .T. ) ;
#8442=CYLINDRICAL_SURFACE ( 'NONE', #4596, 1.999999999999998446 ) ;
#8445=FACE_OUTER_BOUND ( 'NONE', #38, .T. ) ;
#8447=CARTESIAN_POINT ( 'NONE',  ( -6.000000000000000888, 7.347880794884120722E-16, 4.500000000000000888 ) ) ;
#8462=VECTOR ( 'NONE', #13084, 1000.000000000000000 ) ;
#8464=AXIS2_PLACEMENT_3D ( 'NONE', #15178, #9248, #2182 ) ;
#8471=LINE ( 'NONE', #7256, #3503 ) ;
#8478=ORIENTED_EDGE ( 'NONE', *, *, #2575, .F. ) ;
#8483=CARTESIAN_POINT ( 'NONE',  ( 33.82574562093736859, -6.697933970950280091, -2.000000000000000888 ) ) ;
#8489=ORIENTED_EDGE ( 'NONE', *, *, #11899, .T. ) ;
#8525=EDGE_LOOP ( 'NONE', ( #15072, #5663, #5512, #4423, #5856 ) ) ;
#8534=AXIS2_PLACEMENT_3D ( 'NONE', #2733, #14257, #1424 ) ;
#8550=DIRECTION ( 'NONE',  ( -0.000000000000000000, -0.000000000000000000, 1.000000000000000000 ) ) ;
#8567=( NAMED_UNIT ( * ) SI_UNIT ( $, .STERADIAN. ) SOLID_ANGLE_UNIT ( ) );
#8571=CYLINDRICAL_SURFACE ( 'NONE', #7123, 2.999999999999975131 ) ;
#8573=FACE_OUTER_BOUND ( 'NONE', #6083, .T. ) ;
#8578=VECTOR ( 'NONE', #1771, 1000.000000000000114 ) ;
#8612=CARTESIAN_POINT ( 'NONE',  ( 80.82762530298222714, -9.999999999999994671, 4.000000000000003553 ) ) ;
#8619=LINE ( 'NONE', #7556, #8221 ) ;
#8622=VERTEX_POINT ( 'NONE', #5718 ) ;
#8624=CARTESIAN_POINT ( 'NONE',  ( 0.000000000000000000, 0.000000000000000000, 4.500000000000000888 ) ) ;
#8627=CARTESIAN_POINT ( 'NONE',  ( 91.46153288930040048, 16.46030115554384565, -2.000000000000000888 ) ) ;
#8629=EDGE_CURVE ( 'NONE', #12163, #613, #1353, .T. ) ;
#8633=DIRECTION ( 'NONE',  ( -0.4571871344001417481, -0.8893705212896291235, 0.000000000000000000 ) ) ;
#8647=VECTOR ( 'NONE', #11516, 1000.000000000000000 ) ;
#8656=CARTESIAN_POINT ( 'NONE',  ( 80.00000000000000000, 0.000000000000000000, 4.000000000000003553 ) ) ;
#8661=CARTESIAN_POINT ( 'NONE',  ( 67.23404255319145761, 28.93147646537026318, 4.000000000000003553 ) ) ;
#8677=ADVANCED_FACE ( 'NONE', ( #15021 ), #1024, .T. ) ;
#8679=ORIENTED_EDGE ( 'NONE', *, *, #9619, .F. ) ;
#8684=VERTEX_POINT ( 'NONE', #12621 ) ;
#8701=DIRECTION ( 'NONE',  ( 0.9863939238321437486, 0.1643989873053574857, -0.000000000000000000 ) ) ;
#8708=PLANE ( 'NONE',  #4141 ) ;
#8709=EDGE_CURVE ( 'NONE', #3460, #3172, #4308, .T. ) ;
#8711=( NAMED_UNIT ( * ) PLANE_ANGLE_UNIT ( ) SI_UNIT ( $, .RADIAN. ) );
#8714=ADVANCED_FACE ( 'NONE', ( #9101 ), #4720, .F. ) ;
#8734=DIRECTION ( 'NONE',  ( 0.9148936170212768060, 0.4036950204470268200, -0.000000000000000000 ) ) ;
#8735=LINE ( 'NONE', #13430, #13091 ) ;
#8741=ORIENTED_EDGE ( 'NONE', *, *, #9553, .F. ) ;
#8750=CARTESIAN_POINT ( 'NONE',  ( 72.68384697807672978, 11.35494834827056110, 4.000000000000000000 ) ) ;
#8756=LINE ( 'NONE', #2930, #8578 ) ;
#8757=EDGE_CURVE ( 'NONE', #9373, #1519, #11175, .T. ) ;
#8758=ORIENTED_EDGE ( 'NONE', *, *, #5121, .T. ) ;
#8762=UNCERTAINTY_MEASURE_WITH_UNIT (LENGTH_MEASURE( 1.000000000000000082E-05 ), #5206, 'distance_accuracy_value', 'NONE');
#8763=DIRECTION ( 'NONE',  ( 0.000000000000000000, 0.000000000000000000, 1.000000000000000000 ) ) ;
#8787=ORIENTED_EDGE ( 'NONE', *, *, #7895, .T. ) ;
#8807=EDGE_CURVE ( 'NONE', #6626, #6827, #307, .T. ) ;
#8811=CARTESIAN_POINT ( 'NONE',  ( 3.948182771089140175, -23.68909662653485171, 2.000000000000000000 ) ) ;
#8822=CARTESIAN_POINT ( 'NONE',  ( 80.00000000000000000, 0.000000000000000000, 4.000000000000003553 ) ) ;
#8824=ORIENTED_EDGE ( 'NONE', *, *, #11205, .T. ) ;
#8827=DIRECTION ( 'NONE',  ( 1.000000000000000000, 0.000000000000000000, 0.000000000000000000 ) ) ;
#8831=CARTESIAN_POINT ( 'NONE',  ( 62.65957446808508280, 26.91300136313512681, 7.000000000000000000 ) ) ;
#8834=AXIS2_PLACEMENT_3D ( 'NONE', #12275, #3824, #14284 ) ;
#8857=ORIENTED_EDGE ( 'NONE', *, *, #2242, .T. ) ;
#8860=ORIENTED_EDGE ( 'NONE', *, *, #4240, .T. ) ;
#8861=VERTEX_POINT ( 'NONE', #10921 ) ;
#8871=ORIENTED_EDGE ( 'NONE', *, *, #11076, .F. ) ;
#8875=ORIENTED_EDGE ( 'NONE', *, *, #7853, .T. ) ;
#8879=ORIENTED_EDGE ( 'NONE', *, *, #3364, .F. ) ;
#8883=CARTESIAN_POINT ( 'NONE',  ( 93.63799900313688340, -2.337932895214617890, -2.000000000000000888 ) ) ;
#8887=EDGE_CURVE ( 'NONE', #10221, #3461, #7328, .T. ) ;
#8900=ORIENTED_EDGE ( 'NONE', *, *, #14987, .T. ) ;
#8903=CIRCLE ( 'NONE', #14806, 9.999999999999994671 ) ;
#8917=VERTEX_POINT ( 'NONE', #14550 ) ;
#8926=CARTESIAN_POINT ( 'NONE',  ( 56.98919079003883326, 3.953582723775848962, 7.000000000000000000 ) ) ;
#8936=DIRECTION ( 'NONE',  ( 1.000000000000000000, 0.000000000000000000, 0.000000000000000000 ) ) ;
#8948=ADVANCED_FACE ( 'NONE', ( #14778 ), #3943, .F. ) ;
#8954=ORIENTED_EDGE ( 'NONE', *, *, #4440, .F. ) ;
#8957=ORIENTED_EDGE ( 'NONE', *, *, #12834, .T. ) ;
#8960=CARTESIAN_POINT ( 'NONE',  ( 98.33955663538051795, 3.898681236723621879, -2.000000000000000888 ) ) ;
#8962=SHAPE_DEFINITION_REPRESENTATION ( #10326, #1017 ) ;
#8967=CIRCLE ( 'NONE', #9703, 2.999999999999975131 ) ;
#8972=LINE ( 'NONE', #7829, #2498 ) ;
#8973=EDGE_CURVE ( 'NONE', #4472, #4704, #8619, .T. ) ;
#8997=EDGE_CURVE ( 'NONE', #241, #13926, #7862, .T. ) ;
#8998=EDGE_LOOP ( 'NONE', ( #14275, #2896, #14520, #15101 ) ) ;
#8999=ORIENTED_EDGE ( 'NONE', *, *, #14005, .F. ) ;
#9007=MECHANICAL_DESIGN_GEOMETRIC_PRESENTATION_REPRESENTATION('',(#7781),#9997);
#9010=ORIENTED_EDGE ( 'NONE', *, *, #2577, .T. ) ;
#9014=CIRCLE ( 'NONE', #10735, 11.66666666666667318 ) ;
#9016=LINE ( 'NONE', #6784, #5479 ) ;
#9020=VECTOR ( 'NONE', #3495, 1000.000000000000000 ) ;
#9047=CARTESIAN_POINT ( 'NONE',  ( 18.71314632718394222, -23.25585687728512241, 2.000000000000000000 ) ) ;
#9048=VECTOR ( 'NONE', #179, 1000.000000000000114 ) ;
#9055=ORIENTED_EDGE ( 'NONE', *, *, #9748, .T. ) ;
#9057=CARTESIAN_POINT ( 'NONE',  ( 75.20570977803312473, 12.97982004111159959, 7.000000000000000000 ) ) ;
#9063=EDGE_CURVE ( 'NONE', #10155, #14360, #12682, .T. ) ;
#9081=ORIENTED_EDGE ( 'NONE', *, *, #8629, .F. ) ;
#9082=ORIENTED_EDGE ( 'NONE', *, *, #3910, .T. ) ;
#9091=PLANE ( 'NONE',  #12436 ) ;
#9092=CARTESIAN_POINT ( 'NONE',  ( 66.02295749185037721, 31.67615731643408949, 2.000000000000000000 ) ) ;
#9101=FACE_OUTER_BOUND ( 'NONE', #14150, .T. ) ;
#9109=CARTESIAN_POINT ( 'NONE',  ( 15.21482963846748504, 16.90833299098317610, -130.1575142076926852 ) ) ;
#9114=ORIENTED_EDGE ( 'NONE', *, *, #7877, .F. ) ;
#9115=LINE ( 'NONE', #13568, #6314 ) ;
#9119=EDGE_CURVE ( 'NONE', #4384, #2817, #3760, .T. ) ;
#9121=DIRECTION ( 'NONE',  ( -0.9148936170212769170, -0.4036950204470262649, 0.000000000000000000 ) ) ;
#9132=AXIS2_PLACEMENT_3D ( 'NONE', #10649, #101, #4824 ) ;
#9135=CARTESIAN_POINT ( 'NONE',  ( 72.49759028996471955, 17.18292470770558822, -2.000000000000000888 ) ) ;
#9142=LINE ( 'NONE', #15061, #14100 ) ;
#9144=CIRCLE ( 'NONE', #6935, 11.66666666666667318 ) ;
#9146=CARTESIAN_POINT ( 'NONE',  ( 0.04387302227425586565, -0.8988970056815597243, 4.000000000000000000 ) ) ;
#9156=CARTESIAN_POINT ( 'NONE',  ( 98.48580539929344013, 0.9022481406819604643, 4.000000000000000000 ) ) ;
#9173=EDGE_CURVE ( 'NONE', #4864, #3507, #5995, .T. ) ;
#9179=VECTOR ( 'NONE', #7253, 1000.000000000000114 ) ;
#9180=AXIS2_PLACEMENT_3D ( 'NONE', #240, #7769, #10711 ) ;
#9190=VECTOR ( 'NONE', #4534, 1000.000000000000000 ) ;
#9196=CIRCLE ( 'NONE', #2559, 31.62277660168379256 ) ;
#9202=FACE_OUTER_BOUND ( 'NONE', #3028, .T. ) ;
#9203=CARTESIAN_POINT ( 'NONE',  ( 64.00448238961524794, 36.25062540154047497, -2.000000000000000000 ) ) ;
#9210=LINE ( 'NONE', #9135, #9467 ) ;
#9215=EDGE_LOOP ( 'NONE', ( #8441, #7712, #9910, #5587, #818 ) ) ;
#9218=DIRECTION ( 'NONE',  ( 0.000000000000000000, 0.000000000000000000, 1.000000000000000000 ) ) ;
#9219=AXIS2_PLACEMENT_3D ( 'NONE', #10331, #2030, #6715 ) ;
#9221=AXIS2_PLACEMENT_3D ( 'NONE', #7010, #2183, #13782 ) ;
#9227=ORIENTED_EDGE ( 'NONE', *, *, #6087, .F. ) ;
#9240=ORIENTED_EDGE ( 'NONE', *, *, #7895, .F. ) ;
#9248=DIRECTION ( 'NONE',  ( 0.000000000000000000, 0.000000000000000000, 1.000000000000000000 ) ) ;
#9261=DIRECTION ( 'NONE',  ( 0.000000000000000000, 0.000000000000000000, 1.000000000000000000 ) ) ;
#9282=VERTEX_POINT ( 'NONE', #8831 ) ;
#9288=EDGE_CURVE ( 'NONE', #11326, #2590, #6567, .T. ) ;
#9294=ORIENTED_EDGE ( 'NONE', *, *, #5062, .T. ) ;
#9297=CARTESIAN_POINT ( 'NONE',  ( 60.64109936584995353, 31.48746944824151583, -2.000000000000000000 ) ) ;
#9305=ADVANCED_FACE ( 'NONE', ( #13525 ), #13591, .F. ) ;
#9306=ORIENTED_EDGE ( 'NONE', *, *, #7393, .F. ) ;
#9326=DIRECTION ( 'NONE',  ( 0.000000000000000000, 0.000000000000000000, -1.000000000000000000 ) ) ;
#9330=EDGE_CURVE ( 'NONE', #8861, #1742, #1404, .T. ) ;
#9332=AXIS2_PLACEMENT_3D ( 'NONE', #1127, #7042, #12792 ) ;
#9360=DIRECTION ( 'NONE',  ( 0.000000000000000000, 0.000000000000000000, 1.000000000000000000 ) ) ;
#9369=CARTESIAN_POINT ( 'NONE',  ( 93.34550147531103903, 3.654933296868752457, 7.000000000000000000 ) ) ;
#9373=VERTEX_POINT ( 'NONE', #6832 ) ;
#9378=DIRECTION ( 'NONE',  ( 0.000000000000000000, 0.000000000000000000, 1.000000000000000000 ) ) ;
#9384=EDGE_CURVE ( 'NONE', #1181, #5498, #7303, .T. ) ;
#9387=VERTEX_POINT ( 'NONE', #7757 ) ;
#9402=VERTEX_POINT ( 'NONE', #9297 ) ;
#9404=DIRECTION ( 'NONE',  ( 1.000000000000000000, 0.000000000000000000, 0.000000000000000000 ) ) ;
#9415=CYLINDRICAL_SURFACE ( 'NONE', #785, 6.000000000000005329 ) ;
#9423=VECTOR ( 'NONE', #6174, 1000.000000000000000 ) ;
#9429=LINE ( 'NONE', #1445, #2142 ) ;
#9445=ORIENTED_EDGE ( 'NONE', *, *, #15079, .T. ) ;
#9459=EDGE_CURVE ( 'NONE', #2812, #10393, #2065, .T. ) ;
#9467=VECTOR ( 'NONE', #12440, 1000.000000000000000 ) ;
#9468=LINE ( 'NONE', #6016, #10683 ) ;
#9476=DIRECTION ( 'NONE',  ( -0.000000000000000000, -0.000000000000000000, -1.000000000000000000 ) ) ;
#9478=VECTOR ( 'NONE', #1332, 1000.000000000000000 ) ;
#9493=CARTESIAN_POINT ( 'NONE',  ( 72.68384697807672978, 11.35494834827056110, 7.000000000000000000 ) ) ;
#9501=CARTESIAN_POINT ( 'NONE',  ( 76.00000000000000000, 4.898587196589420717E-16, -130.1575142076926852 ) ) ;
#9511=LINE ( 'NONE', #12960, #414 ) ;
#9517=ORIENTED_EDGE ( 'NONE', *, *, #1784, .T. ) ;
#9525=ADVANCED_FACE ( 'NONE', ( #2366 ), #5973, .F. ) ;
#9539=CARTESIAN_POINT ( 'NONE',  ( 56.98919079003883326, 3.953582723775848962, 7.000000000000000000 ) ) ;
#9544=CIRCLE ( 'NONE', #8314, 3.000000000000002665 ) ;
#9548=ORIENTED_EDGE ( 'NONE', *, *, #257, .F. ) ;
#9549=DIRECTION ( 'NONE',  ( -0.9863939238321437486, -0.1643989873053572359, 0.000000000000000000 ) ) ;
#9553=EDGE_CURVE ( 'NONE', #497, #2656, #924, .T. ) ;
#9558=FACE_OUTER_BOUND ( 'NONE', #9838, .T. ) ;
#9565=ORIENTED_EDGE ( 'NONE', *, *, #2204, .T. ) ;
#9570=ADVANCED_FACE ( 'NONE', ( #8200 ), #112, .T. ) ;
#9574=EDGE_CURVE ( 'NONE', #13626, #1861, #12879, .T. ) ;
#9587=CARTESIAN_POINT ( 'NONE',  ( 14.27437366993929579, -27.03703358530833967, 5.000000000000000000 ) ) ;
#9591=DIRECTION ( 'NONE',  ( -0.000000000000000000, -0.000000000000000000, -1.000000000000000000 ) ) ;
#9601=ORIENTED_EDGE ( 'NONE', *, *, #2510, .T. ) ;
#9613=ORIENTED_EDGE ( 'NONE', *, *, #10396, .F. ) ;
#9619=EDGE_CURVE ( 'NONE', #2590, #7147, #9511, .T. ) ;
#9637=ORIENTED_EDGE ( 'NONE', *, *, #437, .F. ) ;
#9640=DIRECTION ( 'NONE',  ( 1.000000000000000000, 0.000000000000000000, 0.000000000000000000 ) ) ;
#9645=CARTESIAN_POINT ( 'NONE',  ( 86.00000000000000000, 0.000000000000000000, 7.000000000000000000 ) ) ;
#9666=DIRECTION ( 'NONE',  ( 1.000000000000000000, 0.000000000000000000, 0.000000000000000000 ) ) ;
#9682=DIRECTION ( 'NONE',  ( 1.000000000000000000, 0.000000000000000000, -0.000000000000000000 ) ) ;
#9683=CYLINDRICAL_SURFACE ( 'NONE', #6984, 2.999999999999988898 ) ;
#9687=VECTOR ( 'NONE', #8633, 1000.000000000000114 ) ;
#9688=DIRECTION ( 'NONE',  ( 1.000000000000000000, 0.000000000000000000, 0.000000000000000000 ) ) ;
#9696=VERTEX_POINT ( 'NONE', #12032 ) ;
#9697=ORIENTED_EDGE ( 'NONE', *, *, #8412, .F. ) ;
#9703=AXIS2_PLACEMENT_3D ( 'NONE', #2736, #2883, #5132 ) ;
#9707=DIRECTION ( 'NONE',  ( 1.000000000000000000, 0.000000000000000000, 0.000000000000000000 ) ) ;
#9717=LINE ( 'NONE', #14119, #9687 ) ;
#9718=ORIENTED_EDGE ( 'NONE', *, *, #11813, .T. ) ;
#9727=FACE_OUTER_BOUND ( 'NONE', #6647, .T. ) ;
#9736=ORIENTED_EDGE ( 'NONE', *, *, #5488, .T. ) ;
#9746=DIRECTION ( 'NONE',  ( -0.4036950204470267645, 0.9148936170212766950, 0.000000000000000000 ) ) ;
#9748=EDGE_CURVE ( 'NONE', #613, #12163, #7811, .T. ) ;
#9751=LINE ( 'NONE', #585, #6828 ) ;
#9757=VECTOR ( 'NONE', #10050, 1000.000000000000114 ) ;
#9767=DIRECTION ( 'NONE',  ( 1.000000000000000000, 0.000000000000000000, 0.000000000000000000 ) ) ;
#9775=LINE ( 'NONE', #8612, #12900 ) ;
#9796=CARTESIAN_POINT ( 'NONE',  ( -9.999999999999992895, -25.00000000000000000, -130.1575142076926852 ) ) ;
#9800=EDGE_LOOP ( 'NONE', ( #7927, #13170, #2460, #12259 ) ) ;
#9803=DIRECTION ( 'NONE',  ( 1.000000000000000000, 0.000000000000000000, -0.000000000000000000 ) ) ;
#9804=SHAPE_REPRESENTATION_RELATIONSHIP ( 'NONE' , 'NONE' ,  #1017, #14434 ) ;
#9809=CARTESIAN_POINT ( 'NONE',  ( 67.23404255319145761, 28.93147646537025963, -8.169391093593850073 ) ) ;
#9826=PLANE ( 'NONE',  #6873 ) ;
#9832=DIRECTION ( 'NONE',  ( 1.000000000000000000, 0.000000000000000000, 0.000000000000000000 ) ) ;
#9835=CARTESIAN_POINT ( 'NONE',  ( -9.999999999999998224, -1.390791565672605534, -130.1575142076926852 ) ) ;
#9838=EDGE_LOOP ( 'NONE', ( #10590, #8860, #6964, #4128 ) ) ;
#9839=DIRECTION ( 'NONE',  ( 1.000000000000000000, 0.000000000000000000, 0.000000000000000000 ) ) ;
#9841=EDGE_CURVE ( 'NONE', #12348, #9402, #10116, .T. ) ;
#9846=ORIENTED_EDGE ( 'NONE', *, *, #10396, .T. ) ;
#9859=CARTESIAN_POINT ( 'NONE',  ( 101.6227766016837819, -9.999999999999994671, -130.1575142076926852 ) ) ;
#9873=ORIENTED_EDGE ( 'NONE', *, *, #7156, .F. ) ;
#9874=DIRECTION ( 'NONE',  ( 2.081668171172168513E-16, -1.000000000000000000, 0.000000000000000000 ) ) ;
#9875=CARTESIAN_POINT ( 'NONE',  ( 91.12964445316929130, 15.08873975234342701, 7.000000000000000000 ) ) ;
#9892=CARTESIAN_POINT ( 'NONE',  ( 72.49759028996473376, 17.18292470770558822, 4.000000000000000000 ) ) ;
#9894=LINE ( 'NONE', #6371, #7724 ) ;
#9898=LINE ( 'NONE', #14599, #12903 ) ;
#9910=ORIENTED_EDGE ( 'NONE', *, *, #9288, .T. ) ;
#9912=CARTESIAN_POINT ( 'NONE',  ( 18.87754531448929995, -24.24225080111726527, 7.000000000000000000 ) ) ;
#9919=AXIS2_PLACEMENT_3D ( 'NONE', #13133, #3844, #10908 ) ;
#9946=FACE_BOUND ( 'NONE', #1452, .T. ) ;
#9947=VECTOR ( 'NONE', #5416, 1000.000000000000227 ) ;
#9948=FILL_AREA_STYLE_COLOUR ( '', #1658 ) ;
#9963=EDGE_CURVE ( 'NONE', #9387, #9402, #14026, .T. ) ;
#9972=AXIS2_PLACEMENT_3D ( 'NONE', #5447, #10118, #14889 ) ;
#9983=ORIENTED_EDGE ( 'NONE', *, *, #11255, .T. ) ;
#9997=( GEOMETRIC_REPRESENTATION_CONTEXT ( 3 ) GLOBAL_UNCERTAINTY_ASSIGNED_CONTEXT ( ( #12763 ) ) GLOBAL_UNIT_ASSIGNED_CONTEXT ( ( #13444, #1763, #6448 ) ) REPRESENTATION_CONTEXT ( 'NONE', 'WORKASPACE' ) );
#10010=LINE ( 'NONE', #7702, #1202 ) ;
#10011=CARTESIAN_POINT ( 'NONE',  ( 18.21994936526786901, -20.29667510578869027, 4.000000000000000000 ) ) ;
#10020=DIRECTION ( 'NONE',  ( -0.4036950204470267645, 0.9148936170212768060, 0.000000000000000000 ) ) ;
#10021=CIRCLE ( 'NONE', #2172, 10.00000000000000000 ) ;
#10042=EDGE_CURVE ( 'NONE', #5604, #11593, #7032, .T. ) ;
#10046=CARTESIAN_POINT ( 'NONE',  ( 65.21556745095632834, 33.50594455047664866, -2.000000000000000000 ) ) ;
#10050=DIRECTION ( 'NONE',  ( 0.9148936170212769170, 0.4036950204470262649, -0.000000000000000000 ) ) ;
#10059=LINE ( 'NONE', #9203, #7161 ) ;
#10067=CARTESIAN_POINT ( 'NONE',  ( 98.48580539929344013, 0.9022481406819604643, -2.000000000000000888 ) ) ;
#10094=CARTESIAN_POINT ( 'NONE',  ( 86.17559721729969624, 12.01344854909570259, 7.000000000000000000 ) ) ;
#10116=LINE ( 'NONE', #1043, #5123 ) ;
#10118=DIRECTION ( 'NONE',  ( -0.000000000000000000, -0.000000000000000000, 1.000000000000000000 ) ) ;
#10127=VECTOR ( 'NONE', #9218, 1000.000000000000000 ) ;
#10131=ADVANCED_FACE ( 'NONE', ( #4033, #11097, #13172, #9946, #1653, #3884, #1499 ), #8708, .F. ) ;
#10155=VERTEX_POINT ( 'NONE', #1568 ) ;
#10165=LINE ( 'NONE', #6641, #291 ) ;
#10186=DIRECTION ( 'NONE',  ( 1.000000000000000000, 0.000000000000000000, 0.000000000000000000 ) ) ;
#10210=ORIENTED_EDGE ( 'NONE', *, *, #4957, .F. ) ;
#10221=VERTEX_POINT ( 'NONE', #11605 ) ;
#10223=DIRECTION ( 'NONE',  ( 0.000000000000000000, 0.000000000000000000, 1.000000000000000000 ) ) ;
#10238=EDGE_CURVE ( 'NONE', #2494, #8331, #3890, .T. ) ;
#10258=CARTESIAN_POINT ( 'NONE',  ( 0.000000000000000000, 0.000000000000000000, 4.500000000000000888 ) ) ;
#10270=ORIENTED_EDGE ( 'NONE', *, *, #7835, .T. ) ;
#10280=CARTESIAN_POINT ( 'NONE',  ( 14.27437366993929579, -27.03703358530833967, -2.000000000000000000 ) ) ;
#10300=FACE_OUTER_BOUND ( 'NONE', #12836, .T. ) ;
#10308=EDGE_CURVE ( 'NONE', #7147, #10776, #5866, .T. ) ;
#10309=ORIENTED_EDGE ( 'NONE', *, *, #4665, .T. ) ;
#10324=ORIENTED_EDGE ( 'NONE', *, *, #14987, .F. ) ;
#10326=PRODUCT_DEFINITION_SHAPE ( 'NONE', 'NONE',  #12070 ) ;
#10330=ADVANCED_FACE ( 'NONE', ( #6153 ), #9683, .F. ) ;
#10331=CARTESIAN_POINT ( 'NONE',  ( 56.98919079003883326, 3.953582723775848962, -2.000000000000000888 ) ) ;
#10345=CARTESIAN_POINT ( 'NONE',  ( 10.00000000000000178, -1.390791565672601315, 4.000000000000003553 ) ) ;
#10366=CIRCLE ( 'NONE', #14300, 1.999999999999998890 ) ;
#10369=EDGE_CURVE ( 'NONE', #4549, #1993, #1538, .T. ) ;
#10382=DIRECTION ( 'NONE',  ( 0.000000000000000000, 0.000000000000000000, 1.000000000000000000 ) ) ;
#10393=VERTEX_POINT ( 'NONE', #5997 ) ;
#10396=EDGE_CURVE ( 'NONE', #13819, #7470, #13351, .T. ) ;
#10399=CLOSED_SHELL ( 'NONE', ( #15068, #2919, #593, #9305, #11522, #2335, #857, #2562, #4766, #11540, #10131, #14054, #7517, #4131, #5931, #5723, #8677, #9570, #12807, #12707, #14286, #6416, #14347, #4496, #11597, #4699, #1474, #13735, #13325, #7565, #5907, #7412, #13861, #4982, #13969, #5442, #6144, #14017, #3048, #14260, #9525, #2980, #1956, #14199, #10330, #7179, #6190, #14758, #4451, #12833, #1179, #8714, #5969, #7411, #11512, #8948 ) ) ;
#10401=CARTESIAN_POINT ( 'NONE',  ( -6.000000000000000888, 7.347880794884120722E-16, 4.500000000000000888 ) ) ;
#10404=CIRCLE ( 'NONE', #1576, 3.000000000000002665 ) ;
#10414=FACE_OUTER_BOUND ( 'NONE', #14848, .T. ) ;
#10422=CARTESIAN_POINT ( 'NONE',  ( 13.94557569532858032, -25.06424573764405395, 7.000000000000000000 ) ) ;
#10427=DIRECTION ( 'NONE',  ( -0.000000000000000000, -0.000000000000000000, 1.000000000000000000 ) ) ;
#10437=ORIENTED_EDGE ( 'NONE', *, *, #13609, .T. ) ;
#10455=AXIS2_PLACEMENT_3D ( 'NONE', #8926, #14715, #12471 ) ;
#10461=DIRECTION ( 'NONE',  ( 0.04874958797097356245, -0.9988110320138942066, 0.000000000000000000 ) ) ;
#10468=LINE ( 'NONE', #12690, #3542 ) ;
#10474=EDGE_LOOP ( 'NONE', ( #14340, #10210, #9565, #10976 ) ) ;
#10482=DIRECTION ( 'NONE',  ( 1.000000000000000000, 0.000000000000000000, 0.000000000000000000 ) ) ;
#10488=LINE ( 'NONE', #15190, #6000 ) ;
#10492=VECTOR ( 'NONE', #43, 1000.000000000000000 ) ;
#10496=ORIENTED_EDGE ( 'NONE', *, *, #11352, .F. ) ;
#10521=EDGE_LOOP ( 'NONE', ( #8787, #9601, #9227, #15198, #7379, #2780, #5787, #3756 ) ) ;
#10529=EDGE_CURVE ( 'NONE', #5666, #2017, #12129, .T. ) ;
#10537=CARTESIAN_POINT ( 'NONE',  ( 64.81187243050929681, 34.42083816749791936, 7.000000000000000000 ) ) ;
#10548=CARTESIAN_POINT ( 'NONE',  ( 60.23740434540291488, 32.40236306526279009, 5.000000000000000888 ) ) ;
#10558=FACE_OUTER_BOUND ( 'NONE', #1060, .T. ) ;
#10565=CARTESIAN_POINT ( 'NONE',  ( 98.48580539929344013, 0.9022481406819604643, 7.000000000000000000 ) ) ;
#10590=ORIENTED_EDGE ( 'NONE', *, *, #9288, .F. ) ;
#10614=EDGE_CURVE ( 'NONE', #6170, #13370, #13824, .T. ) ;
#10623=FACE_OUTER_BOUND ( 'NONE', #7457, .T. ) ;
#10624=CARTESIAN_POINT ( 'NONE',  ( 8.961831343790189308, 9.104486995144791095, -130.1575142076926852 ) ) ;
#10626=ORIENTED_EDGE ( 'NONE', *, *, #7015, .F. ) ;
#10631=DIRECTION ( 'NONE',  ( -0.000000000000000000, -0.000000000000000000, 1.000000000000000000 ) ) ;
#10645=PLANE ( 'NONE',  #9332 ) ;
#10646=ORIENTED_EDGE ( 'NONE', *, *, #3261, .F. ) ;
#10649=CARTESIAN_POINT ( 'NONE',  ( 88.46153288930041469, 16.46030115554384565, 7.000000000000000000 ) ) ;
#10653=ORIENTED_EDGE ( 'NONE', *, *, #1459, .F. ) ;
#10678=CARTESIAN_POINT ( 'NONE',  ( 80.00000000000000000, 0.000000000000000000, -130.1575142076926852 ) ) ;
#10679=ORIENTED_EDGE ( 'NONE', *, *, #9063, .T. ) ;
#10683=VECTOR ( 'NONE', #14165, 1000.000000000000114 ) ;
#10691=EDGE_LOOP ( 'NONE', ( #619, #4246, #9, #7920, #2718, #662, #5184, #9736, #4380, #7633, #13809, #12823, #8824, #4504, #8900, #13993 ) ) ;
#10693=AXIS2_PLACEMENT_3D ( 'NONE', #14684, #4154, #8827 ) ;
#10694=CIRCLE ( 'NONE', #8464, 4.999999999999997335 ) ;
#10696=EDGE_CURVE ( 'NONE', #9402, #12714, #9142, .T. ) ;
#10711=DIRECTION ( 'NONE',  ( 1.000000000000000000, 0.000000000000000000, 0.000000000000000000 ) ) ;
#10714=CARTESIAN_POINT ( 'NONE',  ( 61.44848940674400239, 29.65768221419895667, 4.000000000000000000 ) ) ;
#10729=VERTEX_POINT ( 'NONE', #5619 ) ;
#10735=AXIS2_PLACEMENT_3D ( 'NONE', #13728, #657, #10186 ) ;
#10749=CYLINDRICAL_SURFACE ( 'NONE', #5657, 31.62277660168379256 ) ;
#10757=CIRCLE ( 'NONE', #185, 4.000000000000003553 ) ;
#10766=CARTESIAN_POINT ( 'NONE',  ( 0.000000000000000000, 0.000000000000000000, 4.500000000000000888 ) ) ;
#10776=VERTEX_POINT ( 'NONE', #44 ) ;
#10786=CARTESIAN_POINT ( 'NONE',  ( 8.961831343790189308, 9.104486995144789319, 7.000000000000000000 ) ) ;
#10799=CARTESIAN_POINT ( 'NONE',  ( 0.000000000000000000, 0.000000000000000000, 4.000000000000000000 ) ) ;
#10800=SURFACE_SIDE_STYLE ('',( #5131 ) ) ;
#10801=DIRECTION ( 'NONE',  ( 1.000000000000000000, -6.245004513516508695E-15, 0.000000000000000000 ) ) ;
#10810=ORIENTED_EDGE ( 'NONE', *, *, #11076, .T. ) ;
#10814=DIRECTION ( 'NONE',  ( -0.9148936170212769170, -0.4036950204470268755, 0.000000000000000000 ) ) ;
#10846=DIRECTION ( 'NONE',  ( 1.000000000000000000, 0.000000000000000000, 0.000000000000000000 ) ) ;
#10854=CARTESIAN_POINT ( 'NONE',  ( 67.23404255319145761, 28.93147646537026318, 7.000000000000000000 ) ) ;
#10896=DIRECTION ( 'NONE',  ( -0.000000000000000000, -0.000000000000000000, 1.000000000000000000 ) ) ;
#10899=VECTOR ( 'NONE', #3560, 1000.000000000000000 ) ;
#10904=EDGE_LOOP ( 'NONE', ( #7389, #6719, #12895, #9517 ) ) ;
#10908=DIRECTION ( 'NONE',  ( 1.000000000000000000, 0.000000000000000000, 0.000000000000000000 ) ) ;
#10918=VERTEX_POINT ( 'NONE', #7441 ) ;
#10921=CARTESIAN_POINT ( 'NONE',  ( 4.000000000000000000, 4.898587196589412829E-16, 4.000000000000000000 ) ) ;
#10922=ORIENTED_EDGE ( 'NONE', *, *, #5924, .F. ) ;
#10933=ORIENTED_EDGE ( 'NONE', *, *, #14182, .T. ) ;
#10940=PLANE ( 'NONE',  #8534 ) ;
#10949=CARTESIAN_POINT ( 'NONE',  ( 0.000000000000000000, 0.000000000000000000, 7.000000000000000000 ) ) ;
#10966=DIRECTION ( 'NONE',  ( -0.1643989873053572359, 0.9863939238321437486, 0.000000000000000000 ) ) ;
#10969=CARTESIAN_POINT ( 'NONE',  ( 13.28797974610714761, -21.11867004231547540, -130.1575142076926852 ) ) ;
#10973=CARTESIAN_POINT ( 'NONE',  ( 93.49175023922396122, 0.6585002008270834928, 4.000000000000000000 ) ) ;
#10976=ORIENTED_EDGE ( 'NONE', *, *, #2950, .T. ) ;
#10982=ORIENTED_EDGE ( 'NONE', *, *, #2163, .F. ) ;
#10988=EDGE_CURVE ( 'NONE', #4472, #8917, #13269, .T. ) ;
#10993=AXIS2_PLACEMENT_3D ( 'NONE', #2471, #1302, #3843 ) ;
#11013=LINE ( 'NONE', #8627, #845 ) ;
#11016=DIRECTION ( 'NONE',  ( 0.9863939238321436376, 0.1643989873053573192, 0.000000000000000000 ) ) ;
#11018=CARTESIAN_POINT ( 'NONE',  ( 64.81187243050929681, 34.42083816749791936, 5.000000000000000888 ) ) ;
#11032=PLANE ( 'NONE',  #3891 ) ;
#11033=DIRECTION ( 'NONE',  ( 1.000000000000000000, 0.000000000000000000, 0.000000000000000000 ) ) ;
#11035=CARTESIAN_POINT ( 'NONE',  ( 19.25177984293773648, 7.759396820770405157, 4.000000000000003553 ) ) ;
#11060=VERTEX_POINT ( 'NONE', #7897 ) ;
#11062=DIRECTION ( 'NONE',  ( -0.000000000000000000, -0.000000000000000000, 1.000000000000000000 ) ) ;
#11076=EDGE_CURVE ( 'NONE', #12714, #4008, #4305, .T. ) ;
#11094=ORIENTED_EDGE ( 'NONE', *, *, #13137, .T. ) ;
#11097=FACE_BOUND ( 'NONE', #9215, .T. ) ;
#11160=AXIS2_PLACEMENT_3D ( 'NONE', #3256, #3409, #6941 ) ;
#11174=AXIS2_PLACEMENT_3D ( 'NONE', #2633, #151, #5023 ) ;
#11175=CIRCLE ( 'NONE', #11160, 2.999999999999988898 ) ;
#11203=VERTEX_POINT ( 'NONE', #26 ) ;
#11205=EDGE_CURVE ( 'NONE', #3461, #6683, #6502, .T. ) ;
#11214=CARTESIAN_POINT ( 'NONE',  ( 65.94650549498811642, -33.90026220706953808, 4.000000000000000000 ) ) ;
#11222=AXIS2_PLACEMENT_3D ( 'NONE', #14513, #7515, #6356 ) ;
#11224=LINE ( 'NONE', #9912, #7962 ) ;
#11233=AXIS2_PLACEMENT_3D ( 'NONE', #3425, #178, #4670 ) ;
#11239=EDGE_CURVE ( 'NONE', #7126, #12183, #4315, .T. ) ;
#11255=EDGE_CURVE ( 'NONE', #3709, #1757, #4817, .T. ) ;
#11269=VERTEX_POINT ( 'NONE', #2573 ) ;
#11295=AXIS2_PLACEMENT_3D ( 'NONE', #4284, #1987, #12346 ) ;
#11300=ORIENTED_EDGE ( 'NONE', *, *, #14481, .F. ) ;
#11307=DIRECTION ( 'NONE',  ( 0.000000000000000000, 0.000000000000000000, 1.000000000000000000 ) ) ;
#11316=DIRECTION ( 'NONE',  ( 1.000000000000000000, 0.000000000000000000, 0.000000000000000000 ) ) ;
#11319=CARTESIAN_POINT ( 'NONE',  ( 65.21556745095632834, 33.50594455047664866, 2.000000000000000000 ) ) ;
#11326=VERTEX_POINT ( 'NONE', #6341 ) ;
#11328=DIRECTION ( 'NONE',  ( 1.000000000000000000, 0.000000000000000000, 0.000000000000000000 ) ) ;
#11342=CARTESIAN_POINT ( 'NONE',  ( 93.34550147531103903, 3.654933296868752457, 4.000000000000000000 ) ) ;
#11352=EDGE_CURVE ( 'NONE', #5795, #11474, #8967, .T. ) ;
#11356=EDGE_CURVE ( 'NONE', #3172, #7470, #1500, .T. ) ;
#11363=ORIENTED_EDGE ( 'NONE', *, *, #1916, .F. ) ;
#11388=ORIENTED_EDGE ( 'NONE', *, *, #13390, .F. ) ;
#11393=CYLINDRICAL_SURFACE ( 'NONE', #5303, 6.000000000000000888 ) ;
#11394=AXIS2_PLACEMENT_3D ( 'NONE', #3869, #8550, #14086 ) ;
#11397=CYLINDRICAL_SURFACE ( 'NONE', #12243, 10.00000000000000000 ) ;
#11398=EDGE_LOOP ( 'NONE', ( #5970, #4052, #1512, #1354 ) ) ;
#11414=DIRECTION ( 'NONE',  ( 0.9148936170212769170, 0.4036950204470268755, -0.000000000000000000 ) ) ;
#11440=EDGE_CURVE ( 'NONE', #15071, #3292, #14869, .T. ) ;
#11448=CIRCLE ( 'NONE', #4835, 2.000000000000003109 ) ;
#11474=VERTEX_POINT ( 'NONE', #12702 ) ;
#11480=AXIS2_PLACEMENT_3D ( 'NONE', #137, #9378, #2539 ) ;
#11505=AXIS2_PLACEMENT_3D ( 'NONE', #13806, #11790, #11718 ) ;
#11512=ADVANCED_FACE ( 'NONE', ( #5431 ), #7878, .F. ) ;
#11513=ORIENTED_EDGE ( 'NONE', *, *, #5488, .F. ) ;
#11516=DIRECTION ( 'NONE',  ( -0.000000000000000000, -0.000000000000000000, 1.000000000000000000 ) ) ;
#11520=ORIENTED_EDGE ( 'NONE', *, *, #10988, .T. ) ;
#11522=ADVANCED_FACE ( 'NONE', ( #3334 ), #11393, .F. ) ;
#11527=ORIENTED_EDGE ( 'NONE', *, *, #11812, .T. ) ;
#11533=PLANE ( 'NONE',  #7806 ) ;
#11540=ADVANCED_FACE ( 'NONE', ( #11839 ), #15185, .F. ) ;
#11546=CARTESIAN_POINT ( 'NONE',  ( 0.000000000000000000, 0.000000000000000000, 4.500000000000000888 ) ) ;
#11569=DIRECTION ( 'NONE',  ( 0.000000000000000000, 0.000000000000000000, 1.000000000000000000 ) ) ;
#11576=CIRCLE ( 'NONE', #5228, 1.999999999999998890 ) ;
#11585=EDGE_LOOP ( 'NONE', ( #5719, #6458, #8112, #15022 ) ) ;
#11593=VERTEX_POINT ( 'NONE', #11694 ) ;
#11597=ADVANCED_FACE ( 'NONE', ( #10558 ), #12916, .F. ) ;
#11605=CARTESIAN_POINT ( 'NONE',  ( 18.21994936526786901, -20.29667510578869027, 7.000000000000000000 ) ) ;
#11609=EDGE_CURVE ( 'NONE', #10221, #5235, #9468, .T. ) ;
#11616=ORIENTED_EDGE ( 'NONE', *, *, #8997, .T. ) ;
#11619=LINE ( 'NONE', #4621, #10127 ) ;
#11648=VECTOR ( 'NONE', #2749, 1000.000000000000000 ) ;
#11650=ORIENTED_EDGE ( 'NONE', *, *, #6256, .T. ) ;
#11652=LINE ( 'NONE', #12082, #9478 ) ;
#11673=ORIENTED_EDGE ( 'NONE', *, *, #4293, .F. ) ;
#11677=CARTESIAN_POINT ( 'NONE',  ( 80.00000000000000000, 0.000000000000000000, 7.000000000000000000 ) ) ;
#11691=AXIS2_PLACEMENT_3D ( 'NONE', #9156, #11307, #12537 ) ;
#11694=CARTESIAN_POINT ( 'NONE',  ( 31.51081190520435626, 3.030430839836910639, 7.000000000000000000 ) ) ;
#11706=ORIENTED_EDGE ( 'NONE', *, *, #10238, .F. ) ;
#11718=DIRECTION ( 'NONE',  ( 1.000000000000000000, 0.000000000000000000, 0.000000000000000000 ) ) ;
#11728=VECTOR ( 'NONE', #3998, 999.9999999999998863 ) ;
#11733=ORIENTED_EDGE ( 'NONE', *, *, #9841, .F. ) ;
#11734=VECTOR ( 'NONE', #6033, 1000.000000000000114 ) ;
#11737=DIRECTION ( 'NONE',  ( -0.9863939238321437486, -0.1643989873053572359, 0.000000000000000000 ) ) ;
#11754=ORIENTED_EDGE ( 'NONE', *, *, #10696, .T. ) ;
#11755=ORIENTED_EDGE ( 'NONE', *, *, #10238, .T. ) ;
#11760=FACE_BOUND ( 'NONE', #12914, .T. ) ;
#11790=DIRECTION ( 'NONE',  ( -0.000000000000000000, 0.000000000000000000, 1.000000000000000000 ) ) ;
#11801=EDGE_LOOP ( 'NONE', ( #3828, #14326, #12979, #13913, #11650, #6569, #5183, #11527 ) ) ;
#11812=EDGE_CURVE ( 'NONE', #3507, #10221, #710, .T. ) ;
#11813=EDGE_CURVE ( 'NONE', #13917, #5604, #118, .T. ) ;
#11817=DIRECTION ( 'NONE',  ( 0.000000000000000000, 0.000000000000000000, 1.000000000000000000 ) ) ;
#11829=DIRECTION ( 'NONE',  ( -0.9988110320138940956, -0.04874958797097371510, -0.000000000000000000 ) ) ;
#11832=CARTESIAN_POINT ( 'NONE',  ( 101.4858053992934401, 0.9022481406819604643, 4.000000000000000000 ) ) ;
#11833=AXIS2_PLACEMENT_3D ( 'NONE', #13343, #202, #4921 ) ;
#11839=FACE_OUTER_BOUND ( 'NONE', #324, .T. ) ;
#11846=LINE ( 'NONE', #1191, #5833 ) ;
#11858=EDGE_CURVE ( 'NONE', #154, #2812, #7387, .T. ) ;
#11860=CIRCLE ( 'NONE', #2313, 2.999999999999988898 ) ;
#11871=VECTOR ( 'NONE', #12363, 999.9999999999998863 ) ;
#11874=AXIS2_PLACEMENT_3D ( 'NONE', #8028, #9476, #5730 ) ;
#11877=FACE_OUTER_BOUND ( 'NONE', #14967, .T. ) ;
#11899=EDGE_CURVE ( 'NONE', #4314, #10393, #1530, .T. ) ;
#11908=DIRECTION ( 'NONE',  ( 0.000000000000000000, 0.000000000000000000, 1.000000000000000000 ) ) ;
#11909=AXIS2_PLACEMENT_3D ( 'NONE', #1023, #5717, #12911 ) ;
#11916=MECHANICAL_DESIGN_GEOMETRIC_PRESENTATION_REPRESENTATION('',(#14925),#14682);
#11924=DIRECTION ( 'NONE',  ( -0.04874958797097372204, 0.9988110320138942066, 0.000000000000000000 ) ) ;
#11935=FACE_OUTER_BOUND ( 'NONE', #10691, .T. ) ;
#11937=AXIS2_PLACEMENT_3D ( 'NONE', #4221, #14985, #8055 ) ;
#11938=CARTESIAN_POINT ( 'NONE',  ( 0.000000000000000000, 0.000000000000000000, 4.000000000000000000 ) ) ;
#11943=ORIENTED_EDGE ( 'NONE', *, *, #1223, .T. ) ;
#11946=CARTESIAN_POINT ( 'NONE',  ( 88.46153288930041469, 16.46030115554384565, -2.000000000000000888 ) ) ;
#11948=ORIENTED_EDGE ( 'NONE', *, *, #11858, .F. ) ;
#11955=DIRECTION ( 'NONE',  ( 1.000000000000000000, 0.000000000000000000, 0.000000000000000000 ) ) ;
#11956=EDGE_CURVE ( 'NONE', #7258, #11060, #8237, .T. ) ;
#11957=AXIS2_PLACEMENT_3D ( 'NONE', #9092, #13777, #7602 ) ;
#11965=VERTEX_POINT ( 'NONE', #13213 ) ;
#11967=DIRECTION ( 'NONE',  ( -0.4036950204470283188, 0.9148936170212761398, 0.000000000000000000 ) ) ;
#11968=AXIS2_PLACEMENT_3D ( 'NONE', #1335, #6032, #9404 ) ;
#11986=VERTEX_POINT ( 'NONE', #12519 ) ;
#12005=DIRECTION ( 'NONE',  ( -0.000000000000000000, -0.000000000000000000, 1.000000000000000000 ) ) ;
#12025=CARTESIAN_POINT ( 'NONE',  ( 31.51081190520435626, 3.030430839836910639, -2.000000000000000888 ) ) ;
#12026=DIRECTION ( 'NONE',  ( -0.000000000000000000, -0.000000000000000000, -1.000000000000000000 ) ) ;
#12031=CARTESIAN_POINT ( 'NONE',  ( 79.18363542992865689, -10.13606076167855541, 7.000000000000006217 ) ) ;
#12032=CARTESIAN_POINT ( 'NONE',  ( 13.28797974610714761, -21.11867004231547540, 4.000000000000003553 ) ) ;
#12039=CARTESIAN_POINT ( 'NONE',  ( 80.00000000000000000, 0.000000000000000000, -130.1575142076926852 ) ) ;
#12046=ORIENTED_EDGE ( 'NONE', *, *, #7128, .F. ) ;
#12051=ORIENTED_EDGE ( 'NONE', *, *, #12743, .F. ) ;
#12054=CARTESIAN_POINT ( 'NONE',  ( 0.000000000000000000, 0.000000000000000000, 7.000000000000000000 ) ) ;
#12058=ORIENTED_EDGE ( 'NONE', *, *, #6765, .F. ) ;
#12060=EDGE_CURVE ( 'NONE', #7147, #9373, #9210, .T. ) ;
#12067=ORIENTED_EDGE ( 'NONE', *, *, #13814, .F. ) ;
#12070=PRODUCT_DEFINITION ( 'UNKNOWN', '', #2057, #2716 ) ;
#12079=FACE_OUTER_BOUND ( 'NONE', #13688, .T. ) ;
#12080=CARTESIAN_POINT ( 'NONE',  ( 33.82574562093736859, -6.697933970950280091, 4.000000000000000000 ) ) ;
#12082=CARTESIAN_POINT ( 'NONE',  ( 6.000000000000000888, 0.000000000000000000, 4.500000000000000888 ) ) ;
#12088=CARTESIAN_POINT ( 'NONE',  ( 76.00000000000000000, 4.898587196589422689E-16, 4.000000000000003553 ) ) ;
#12097=DIRECTION ( 'NONE',  ( -0.9863939238321437486, -0.1643989873053574857, 0.000000000000000000 ) ) ;
#12110=CARTESIAN_POINT ( 'NONE',  ( 98.63205416320636232, -2.094184955359748468, 4.000000000000000000 ) ) ;
#12129=LINE ( 'NONE', #4232, #11871 ) ;
#12134=DIRECTION ( 'NONE',  ( 0.000000000000000000, 0.000000000000000000, 1.000000000000000000 ) ) ;
#12136=ORIENTED_EDGE ( 'NONE', *, *, #7015, .T. ) ;
#12147=EDGE_CURVE ( 'NONE', #10776, #8684, #5005, .T. ) ;
#12163=VERTEX_POINT ( 'NONE', #2920 ) ;
#12166=DIRECTION ( 'NONE',  ( 0.000000000000000000, 0.000000000000000000, 1.000000000000000000 ) ) ;
#12168=CARTESIAN_POINT ( 'NONE',  ( 86.00000000000000000, 0.000000000000000000, 4.500000000000000888 ) ) ;
#12175=CARTESIAN_POINT ( 'NONE',  ( -9.999999999999998224, 0.000000000000000000, 4.000000000000003553 ) ) ;
#12178=DIRECTION ( 'NONE',  ( -0.000000000000000000, -0.000000000000000000, 1.000000000000000000 ) ) ;
#12183=VERTEX_POINT ( 'NONE', #514 ) ;
#12187=CIRCLE ( 'NONE', #13158, 4.999999999999997335 ) ;
#12199=DIRECTION ( 'NONE',  ( -0.000000000000000000, -0.000000000000000000, -1.000000000000000000 ) ) ;
#12202=EDGE_CURVE ( 'NONE', #2590, #12183, #9898, .T. ) ;
#12206=AXIS2_PLACEMENT_3D ( 'NONE', #8811, #14354, #2972 ) ;
#12217=LINE ( 'NONE', #11214, #11728 ) ;
#12219=CARTESIAN_POINT ( 'NONE',  ( 80.00000000000000000, 0.000000000000000000, 7.000000000000000000 ) ) ;
#12221=AXIS2_PLACEMENT_3D ( 'NONE', #12054, #1, #1385 ) ;
#12231=EDGE_LOOP ( 'NONE', ( #363, #5115 ) ) ;
#12243=AXIS2_PLACEMENT_3D ( 'NONE', #9109, #4121, #11328 ) ;
#12251=ORIENTED_EDGE ( 'NONE', *, *, #12834, .F. ) ;
#12259=ORIENTED_EDGE ( 'NONE', *, *, #13760, .F. ) ;
#12261=DIRECTION ( 'NONE',  ( 1.000000000000000000, 0.000000000000000000, 0.000000000000000000 ) ) ;
#12266=VERTEX_POINT ( 'NONE', #5609 ) ;
#12275=CARTESIAN_POINT ( 'NONE',  ( 80.00000000000000000, 0.000000000000000000, 4.500000000000000888 ) ) ;
#12290=DIRECTION ( 'NONE',  ( 0.000000000000000000, 0.000000000000000000, 1.000000000000000000 ) ) ;
#12300=DIRECTION ( 'NONE',  ( -0.000000000000000000, -0.000000000000000000, 1.000000000000000000 ) ) ;
#12335=AXIS2_PLACEMENT_3D ( 'NONE', #9796, #3789, #11016 ) ;
#12337=ORIENTED_EDGE ( 'NONE', *, *, #12667, .F. ) ;
#12346=DIRECTION ( 'NONE',  ( 1.000000000000000000, 0.000000000000000000, 0.000000000000000000 ) ) ;
#12348=VERTEX_POINT ( 'NONE', #14988 ) ;
#12363=DIRECTION ( 'NONE',  ( 0.4036950204470267645, -0.9148936170212768060, 0.000000000000000000 ) ) ;
#12373=ORIENTED_EDGE ( 'NONE', *, *, #4133, .F. ) ;
#12376=ORIENTED_EDGE ( 'NONE', *, *, #11239, .F. ) ;
#12384=CIRCLE ( 'NONE', #13102, 3.000000000000002665 ) ;
#12388=VERTEX_POINT ( 'NONE', #3368 ) ;
#12397=EDGE_LOOP ( 'NONE', ( #825, #6727, #7192, #6353 ) ) ;
#12407=EDGE_LOOP ( 'NONE', ( #9114, #10496, #21, #11755 ) ) ;
#12411=CARTESIAN_POINT ( 'NONE',  ( 13.45237873341251067, -22.10506396614762537, 2.000000000000000000 ) ) ;
#12413=VECTOR ( 'NONE', #6298, 1000.000000000000000 ) ;
#12420=EDGE_CURVE ( 'NONE', #11060, #7248, #8057, .T. ) ;
#12422=FACE_OUTER_BOUND ( 'NONE', #1367, .T. ) ;
#12436=AXIS2_PLACEMENT_3D ( 'NONE', #8156, #1309, #14235 ) ;
#12437=ORIENTED_EDGE ( 'NONE', *, *, #2396, .F. ) ;
#12440=DIRECTION ( 'NONE',  ( -0.000000000000000000, -0.000000000000000000, 1.000000000000000000 ) ) ;
#12460=ORIENTED_EDGE ( 'NONE', *, *, #6765, .T. ) ;
#12468=AXIS2_PLACEMENT_3D ( 'NONE', #7516, #5150, #3905 ) ;
#12469=VECTOR ( 'NONE', #4101, 1000.000000000000000 ) ;
#12471=DIRECTION ( 'NONE',  ( 1.000000000000000000, 0.000000000000000000, 0.000000000000000000 ) ) ;
#12474=LINE ( 'NONE', #9859, #12469 ) ;
#12480=AXIS2_PLACEMENT_3D ( 'NONE', #800, #3038, #652 ) ;
#12485=EDGE_LOOP ( 'NONE', ( #12373, #1328, #10324, #14223 ) ) ;
#12503=EDGE_CURVE ( 'NONE', #13379, #3242, #11652, .T. ) ;
#12516=CARTESIAN_POINT ( 'NONE',  ( 79.18363542992867110, -10.13606076167855008, 7.000000000000000000 ) ) ;
#12519=CARTESIAN_POINT ( 'NONE',  ( 80.82762530298222714, -9.999999999999994671, 4.000000000000003553 ) ) ;
#12537=DIRECTION ( 'NONE',  ( 1.000000000000000000, 0.000000000000000000, 0.000000000000000000 ) ) ;
#12538=CARTESIAN_POINT ( 'NONE',  ( 3.321103546710217902, -13.95673088054953759, 4.000000000000000000 ) ) ;
#12547=DIRECTION ( 'NONE',  ( -0.000000000000000000, -0.000000000000000000, 1.000000000000000000 ) ) ;
#12589=ORIENTED_EDGE ( 'NONE', *, *, #2587, .F. ) ;
#12616=AXIS2_PLACEMENT_3D ( 'NONE', #12219, #2619, #7315 ) ;
#12621=CARTESIAN_POINT ( 'NONE',  ( 70.16198417812034904, 9.730076655429538590, 4.000000000000000000 ) ) ;
#12634=EDGE_CURVE ( 'NONE', #5235, #13626, #2625, .T. ) ;
#12667=EDGE_CURVE ( 'NONE', #10918, #12266, #13161, .T. ) ;
#12668=EDGE_CURVE ( 'NONE', #14957, #1993, #13627, .T. ) ;
#12669=VERTEX_POINT ( 'NONE', #11319 ) ;
#12682=LINE ( 'NONE', #6998, #6105 ) ;
#12689=AXIS2_PLACEMENT_3D ( 'NONE', #8750, #7539, #7680 ) ;
#12690=CARTESIAN_POINT ( 'NONE',  ( 67.23404255319148604, 28.93147646537027384, 7.000000000000000000 ) ) ;
#12696=FACE_OUTER_BOUND ( 'NONE', #1533, .T. ) ;
#12702=CARTESIAN_POINT ( 'NONE',  ( 91.46153288930040048, 16.46030115554384565, 4.000000000000000000 ) ) ;
#12707=ADVANCED_FACE ( 'NONE', ( #3408 ), #12770, .F. ) ;
#12708=LINE ( 'NONE', #10401, #2076 ) ;
#12709=CARTESIAN_POINT ( 'NONE',  ( 18.71314632718394222, -23.25585687728512241, -2.000000000000000000 ) ) ;
#12714=VERTEX_POINT ( 'NONE', #4565 ) ;
#12716=CYLINDRICAL_SURFACE ( 'NONE', #11968, 6.000000000000005329 ) ;
#12739=ORIENTED_EDGE ( 'NONE', *, *, #4587, .F. ) ;
#12743=EDGE_CURVE ( 'NONE', #12163, #1742, #6709, .T. ) ;
#12763=UNCERTAINTY_MEASURE_WITH_UNIT (LENGTH_MEASURE( 1.000000000000000082E-05 ), #13444, 'distance_accuracy_value', 'NONE');
#12767=EDGE_CURVE ( 'NONE', #13926, #7258, #10694, .T. ) ;
#12770=CYLINDRICAL_SURFACE ( 'NONE', #14870, 9.999999999999994671 ) ;
#12772=DIRECTION ( 'NONE',  ( 1.000000000000000000, 0.000000000000000000, 0.000000000000000000 ) ) ;
#12792=DIRECTION ( 'NONE',  ( 1.000000000000000000, 0.000000000000000000, -0.000000000000000000 ) ) ;
#12807=ADVANCED_FACE ( 'NONE', ( #12696 ), #6868, .T. ) ;
#12811=AXIS2_PLACEMENT_3D ( 'NONE', #919, #4537, #5403 ) ;
#12818=CARTESIAN_POINT ( 'NONE',  ( 18.38434835257323030, -21.28306902962084024, 4.000000000000000000 ) ) ;
#12823=ORIENTED_EDGE ( 'NONE', *, *, #8887, .T. ) ;
#12833=ADVANCED_FACE ( 'NONE', ( #10623 ), #13145, .F. ) ;
#12834=EDGE_CURVE ( 'NONE', #3292, #11269, #5938, .T. ) ;
#12836=EDGE_LOOP ( 'NONE', ( #7429, #2969, #2338, #4892 ) ) ;
#12841=DIRECTION ( 'NONE',  ( 0.000000000000000000, 0.000000000000000000, 1.000000000000000000 ) ) ;
#12847=CARTESIAN_POINT ( 'NONE',  ( -10.00000000000000000, -2.081668171172168513E-15, 7.000000000000000000 ) ) ;
#12862=VECTOR ( 'NONE', #7068, 1000.000000000000114 ) ;
#12864=DIRECTION ( 'NONE',  ( 1.000000000000000000, 0.000000000000000000, 0.000000000000000000 ) ) ;
#12865=DIRECTION ( 'NONE',  ( 0.1643989873053574580, -0.9863939238321436376, 0.000000000000000000 ) ) ;
#12879=LINE ( 'NONE', #9587, #1418 ) ;
#12895=ORIENTED_EDGE ( 'NONE', *, *, #3365, .F. ) ;
#12898=CARTESIAN_POINT ( 'NONE',  ( 60.64109936584995353, 31.48746944824151583, 2.000000000000000000 ) ) ;
#12900=VECTOR ( 'NONE', #6537, 1000.000000000000000 ) ;
#12901=DIRECTION ( 'NONE',  ( -0.9148936170212770280, -0.4036950204470263204, 0.000000000000000000 ) ) ;
#12903=VECTOR ( 'NONE', #4068, 1000.000000000000000 ) ;
#12911=DIRECTION ( 'NONE',  ( 1.000000000000000000, 0.000000000000000000, 0.000000000000000000 ) ) ;
#12914=EDGE_LOOP ( 'NONE', ( #9081, #13008 ) ) ;
#12916=PLANE ( 'NONE',  #2342 ) ;
#12919=EDGE_LOOP ( 'NONE', ( #1692, #8415, #15115, #7375 ) ) ;
#12921=EDGE_CURVE ( 'NONE', #7248, #241, #13872, .T. ) ;
#12927=ORIENTED_EDGE ( 'NONE', *, *, #9459, .F. ) ;
#12960=CARTESIAN_POINT ( 'NONE',  ( 59.05334708265789345, 38.04890259842303379, 4.000000000000000000 ) ) ;
#12975=ORIENTED_EDGE ( 'NONE', *, *, #3261, .T. ) ;
#12979=ORIENTED_EDGE ( 'NONE', *, *, #3209, .F. ) ;
#12981=CARTESIAN_POINT ( 'NONE',  ( 19.20634328910001543, -26.21503864878155099, -2.000000000000000000 ) ) ;
#12989=ORIENTED_EDGE ( 'NONE', *, *, #4440, .T. ) ;
#13008=ORIENTED_EDGE ( 'NONE', *, *, #9748, .F. ) ;
#13010=FACE_BOUND ( 'NONE', #14040, .T. ) ;
#13014=DIRECTION ( 'NONE',  ( -0.000000000000000000, -0.000000000000000000, -1.000000000000000000 ) ) ;
#13034=LINE ( 'NONE', #6836, #8647 ) ;
#13049=AXIS2_PLACEMENT_3D ( 'NONE', #10949, #12026, #2668 ) ;
#13070=CARTESIAN_POINT ( 'NONE',  ( 93.34550147531103903, 3.654933296868752457, -2.000000000000000888 ) ) ;
#13084=DIRECTION ( 'NONE',  ( -0.000000000000000000, -0.000000000000000000, 1.000000000000000000 ) ) ;
#13091=VECTOR ( 'NONE', #14015, 1000.000000000000000 ) ;
#13097=ORIENTED_EDGE ( 'NONE', *, *, #4189, .T. ) ;
#13102=AXIS2_PLACEMENT_3D ( 'NONE', #3753, #11817, #3681 ) ;
#13122=ORIENTED_EDGE ( 'NONE', *, *, #2967, .F. ) ;
#13127=ORIENTED_EDGE ( 'NONE', *, *, #14313, .T. ) ;
#13128=CARTESIAN_POINT ( 'NONE',  ( 18.87754531448929995, -24.24225080111726527, 5.000000000000000000 ) ) ;
#13133=CARTESIAN_POINT ( 'NONE',  ( 80.00000000000000000, 0.000000000000000000, 7.000000000000000000 ) ) ;
#13137=EDGE_CURVE ( 'NONE', #1510, #2255, #3371, .T. ) ;
#13145=PLANE ( 'NONE',  #11174 ) ;
#13158=AXIS2_PLACEMENT_3D ( 'NONE', #9539, #11908, #65 ) ;
#13161=CIRCLE ( 'NONE', #6549, 2.999999999999988898 ) ;
#13162=DIRECTION ( 'NONE',  ( -0.000000000000000000, -0.000000000000000000, 1.000000000000000000 ) ) ;
#13167=ORIENTED_EDGE ( 'NONE', *, *, #5136, .F. ) ;
#13170=ORIENTED_EDGE ( 'NONE', *, *, #1758, .F. ) ;
#13172=FACE_BOUND ( 'NONE', #7435, .T. ) ;
#13178=FACE_OUTER_BOUND ( 'NONE', #12407, .T. ) ;
#13181=FACE_OUTER_BOUND ( 'NONE', #6149, .T. ) ;
#13183=VECTOR ( 'NONE', #8370, 1000.000000000000114 ) ;
#13189=VECTOR ( 'NONE', #4737, 1000.000000000000000 ) ;
#13194=CIRCLE ( 'NONE', #14687, 6.000000000000000888 ) ;
#13204=CARTESIAN_POINT ( 'NONE',  ( 15.21482963846748504, 16.90833299098317610, 7.000000000000006217 ) ) ;
#13213=CARTESIAN_POINT ( 'NONE',  ( 88.84370878116858705, 10.64188714589527507, 4.000000000000000000 ) ) ;
#13217=LINE ( 'NONE', #449, #14410 ) ;
#13248=CARTESIAN_POINT ( 'NONE',  ( 1.006169830977205581, -4.228366069762346413, 4.000000000000000000 ) ) ;
#13268=CARTESIAN_POINT ( 'NONE',  ( 80.82762530298222714, -19.99999999999999645, 4.000000000000003553 ) ) ;
#13269=LINE ( 'NONE', #8883, #11648 ) ;
#13297=CIRCLE ( 'NONE', #9132, 2.999999999999975131 ) ;
#13308=AXIS2_PLACEMENT_3D ( 'NONE', #3980, #10966, #2521 ) ;
#13313=CARTESIAN_POINT ( 'NONE',  ( 14.27437366993929579, -27.03703358530833967, 4.000000000000000000 ) ) ;
#13325=ADVANCED_FACE ( 'NONE', ( #4775 ), #8442, .T. ) ;
#13330=FACE_OUTER_BOUND ( 'NONE', #13513, .T. ) ;
#13340=CARTESIAN_POINT ( 'NONE',  ( 66.02295749185039142, 31.67615731643408949, 4.000000000000000000 ) ) ;
#13343=CARTESIAN_POINT ( 'NONE',  ( 0.000000000000000000, 0.000000000000000000, 7.000000000000000000 ) ) ;
#13349=CARTESIAN_POINT ( 'NONE',  ( 75.68384697807671557, 11.35494834827056110, 7.000000000000000000 ) ) ;
#13351=CIRCLE ( 'NONE', #9919, 6.000000000000005329 ) ;
#13370=VERTEX_POINT ( 'NONE', #3841 ) ;
#13376=VECTOR ( 'NONE', #6926, 1000.000000000000114 ) ;
#13378=ORIENTED_EDGE ( 'NONE', *, *, #4742, .T. ) ;
#13379=VERTEX_POINT ( 'NONE', #2992 ) ;
#13381=CARTESIAN_POINT ( 'NONE',  ( 33.82574562093736859, -6.697933970950280091, -2.000000000000000888 ) ) ;
#13385=ORIENTED_EDGE ( 'NONE', *, *, #437, .T. ) ;
#13390=EDGE_CURVE ( 'NONE', #613, #8861, #13217, .T. ) ;
#13393=MANIFOLD_SOLID_BREP ( 'Cut-Extrude2', #10399 ) ;
#13396=VECTOR ( 'NONE', #4252, 1000.000000000000000 ) ;
#13420=CARTESIAN_POINT ( 'NONE',  ( 74.00000000000000000, 7.347880794884117764E-16, 7.000000000000000000 ) ) ;
#13430=CARTESIAN_POINT ( 'NONE',  ( 74.00000000000000000, 7.347880794884121708E-16, 4.500000000000000888 ) ) ;
#13444=( LENGTH_UNIT ( ) NAMED_UNIT ( * ) SI_UNIT ( .MILLI., .METRE. ) );
#13462=AXIS2_PLACEMENT_3D ( 'NONE', #5173, #12290, #9839 ) ;
#13469=ORIENTED_EDGE ( 'NONE', *, *, #2163, .T. ) ;
#13472=DIRECTION ( 'NONE',  ( 0.4036950204470268200, -0.9148936170212768060, 0.000000000000000000 ) ) ;
#13479=DIRECTION ( 'NONE',  ( 0.1643989873053570416, -0.9863939238321438596, 0.000000000000000000 ) ) ;
#13487=FILL_AREA_STYLE ('',( #9948 ) ) ;
#13499=ORIENTED_EDGE ( 'NONE', *, *, #257, .T. ) ;
#13500=AXIS2_PLACEMENT_3D ( 'NONE', #3747, #7598, #4997 ) ;
#13513=EDGE_LOOP ( 'NONE', ( #3370, #2705, #3526, #12051 ) ) ;
#13525=FACE_OUTER_BOUND ( 'NONE', #11398, .T. ) ;
#13533=DIRECTION ( 'NONE',  ( 1.000000000000000000, 0.000000000000000000, 0.000000000000000000 ) ) ;
#13564=ORIENTED_EDGE ( 'NONE', *, *, #9173, .F. ) ;
#13568=CARTESIAN_POINT ( 'NONE',  ( 70.16198417812034904, 9.730076655429538590, 7.000000000000000000 ) ) ;
#13581=CARTESIAN_POINT ( 'NONE',  ( 83.50748565343083385, 13.38500995229612478, -2.000000000000000888 ) ) ;
#13591=CYLINDRICAL_SURFACE ( 'NONE', #13687, 3.000000000000002665 ) ;
#13603=FACE_OUTER_BOUND ( 'NONE', #265, .T. ) ;
#13609=EDGE_CURVE ( 'NONE', #12348, #2656, #5912, .T. ) ;
#13623=CARTESIAN_POINT ( 'NONE',  ( 62.65957446808508280, 26.91300136313512326, 4.000000000000001776 ) ) ;
#13626=VERTEX_POINT ( 'NONE', #14203 ) ;
#13627=LINE ( 'NONE', #3108, #15151 ) ;
#13631=AXIS2_PLACEMENT_3D ( 'NONE', #3413, #12841, #10482 ) ;
#13636=ORIENTED_EDGE ( 'NONE', *, *, #4509, .F. ) ;
#13651=DIRECTION ( 'NONE',  ( -0.000000000000000000, -0.000000000000000000, 1.000000000000000000 ) ) ;
#13659=PLANE ( 'NONE',  #2180 ) ;
#13671=AXIS2_PLACEMENT_3D ( 'NONE', #7821, #2121, #6593 ) ;
#13681=CARTESIAN_POINT ( 'NONE',  ( 93.63799900313688340, -2.337932895214617890, 4.000000000000000000 ) ) ;
#13687=AXIS2_PLACEMENT_3D ( 'NONE', #10067, #11062, #7460 ) ;
#13688=EDGE_LOOP ( 'NONE', ( #7150, #13564, #5026, #13798 ) ) ;
#13698=AXIS2_PLACEMENT_3D ( 'NONE', #10766, #1468, #9682 ) ;
#13699=AXIS2_PLACEMENT_3D ( 'NONE', #3741, #7202, #2449 ) ;
#13728=CARTESIAN_POINT ( 'NONE',  ( 1.666666666666673624, 0.000000000000000000, 4.000000000000003553 ) ) ;
#13735=ADVANCED_FACE ( 'NONE', ( #1513 ), #5217, .F. ) ;
#13740=ORIENTED_EDGE ( 'NONE', *, *, #3814, .F. ) ;
#13752=DIRECTION ( 'NONE',  ( 2.081668171172168513E-16, -1.000000000000000000, 0.000000000000000000 ) ) ;
#13760=EDGE_CURVE ( 'NONE', #4864, #3461, #3816, .T. ) ;
#13777=DIRECTION ( 'NONE',  ( -0.9148936170212769170, -0.4036950204470268200, 0.000000000000000000 ) ) ;
#13778=CARTESIAN_POINT ( 'NONE',  ( -9.999999999999998224, -1.390791565672605534, 4.000000000000003553 ) ) ;
#13782=DIRECTION ( 'NONE',  ( -0.5416238976136773520, 0.8406209333187989463, 0.000000000000000000 ) ) ;
#13789=EDGE_LOOP ( 'NONE', ( #13378, #5943, #5453, #12739 ) ) ;
#13798=ORIENTED_EDGE ( 'NONE', *, *, #8887, .F. ) ;
#13806=CARTESIAN_POINT ( 'NONE',  ( 0.000000000000000000, 0.000000000000000000, -2.000000000000000000 ) ) ;
#13809=ORIENTED_EDGE ( 'NONE', *, *, #11609, .F. ) ;
#13814=EDGE_CURVE ( 'NONE', #6827, #3709, #1166, .T. ) ;
#13819=VERTEX_POINT ( 'NONE', #13420 ) ;
#13821=DIRECTION ( 'NONE',  ( -0.000000000000000000, -0.000000000000000000, -1.000000000000000000 ) ) ;
#13824=LINE ( 'NONE', #14833, #9190 ) ;
#13827=CYLINDRICAL_SURFACE ( 'NONE', #12811, 2.999999999999988898 ) ;
#13850=VECTOR ( 'NONE', #4846, 1000.000000000000000 ) ;
#13855=ORIENTED_EDGE ( 'NONE', *, *, #12420, .T. ) ;
#13856=CARTESIAN_POINT ( 'NONE',  ( 18.38434835257323030, -21.28306902962084024, 2.000000000000000000 ) ) ;
#13858=VECTOR ( 'NONE', #1717, 1000.000000000000227 ) ;
#13861=ADVANCED_FACE ( 'NONE', ( #744 ), #4438, .F. ) ;
#13872=CIRCLE ( 'NONE', #1115, 4.999999999999997335 ) ;
#13880=FACE_OUTER_BOUND ( 'NONE', #14897, .T. ) ;
#13913=ORIENTED_EDGE ( 'NONE', *, *, #9119, .T. ) ;
#13917=VERTEX_POINT ( 'NONE', #3272 ) ;
#13926=VERTEX_POINT ( 'NONE', #4278 ) ;
#13929=CARTESIAN_POINT ( 'NONE',  ( 19.20634328910001543, -26.21503864878155099, -2.000000000000000000 ) ) ;
#13936=AXIS2_PLACEMENT_3D ( 'NONE', #1142, #9360, #11955 ) ;
#13944=CIRCLE ( 'NONE', #12221, 6.000000000000000888 ) ;
#13963=CIRCLE ( 'NONE', #7580, 2.999999999999988898 ) ;
#13964=DIRECTION ( 'NONE',  ( -0.000000000000000000, -0.000000000000000000, -1.000000000000000000 ) ) ;
#13967=ORIENTED_EDGE ( 'NONE', *, *, #10369, .T. ) ;
#13969=ADVANCED_FACE ( 'NONE', ( #10414 ), #15199, .F. ) ;
#13990=CARTESIAN_POINT ( 'NONE',  ( 65.21556745095632834, 33.50594455047664866, -2.000000000000000000 ) ) ;
#13993=ORIENTED_EDGE ( 'NONE', *, *, #8095, .T. ) ;
#13999=DIRECTION ( 'NONE',  ( 0.000000000000000000, 0.000000000000000000, 1.000000000000000000 ) ) ;
#14005=EDGE_CURVE ( 'NONE', #13926, #12388, #7112, .T. ) ;
#14015=DIRECTION ( 'NONE',  ( -0.000000000000000000, -0.000000000000000000, 1.000000000000000000 ) ) ;
#14017=ADVANCED_FACE ( 'NONE', ( #5738 ), #12716, .F. ) ;
#14026=LINE ( 'NONE', #3494, #11734 ) ;
#14028=DIRECTION ( 'NONE',  ( 0.000000000000000000, 0.000000000000000000, 1.000000000000000000 ) ) ;
#14040=EDGE_LOOP ( 'NONE', ( #10646, #3249, #7367, #2636, #2115 ) ) ;
#14042=ORIENTED_EDGE ( 'NONE', *, *, #7128, .T. ) ;
#14054=ADVANCED_FACE ( 'NONE', ( #14184, #3648, #8334, #13010, #5204, #3796, #11935 ), #10940, .T. ) ;
#14060=VERTEX_POINT ( 'NONE', #12088 ) ;
#14067=PLANE ( 'NONE',  #13698 ) ;
#14068=CARTESIAN_POINT ( 'NONE',  ( 69.97572749000833880, 15.55805301486455683, 4.000000000000000000 ) ) ;
#14086=DIRECTION ( 'NONE',  ( 1.000000000000000000, 0.000000000000000000, 0.000000000000000000 ) ) ;
#14091=CARTESIAN_POINT ( 'NONE',  ( 80.00000000000000000, -9.999999999999994671, 4.000000000000003553 ) ) ;
#14100=VECTOR ( 'NONE', #3448, 1000.000000000000000 ) ;
#14110=DIRECTION ( 'NONE',  ( 1.000000000000000000, 0.000000000000000000, 0.000000000000000000 ) ) ;
#14117=AXIS2_PLACEMENT_3D ( 'NONE', #2253, #3330, #8015 ) ;
#14119=CARTESIAN_POINT ( 'NONE',  ( 60.61028236725008611, -31.15713940066886067, 4.000000000000000000 ) ) ;
#14123=DIRECTION ( 'NONE',  ( 0.4571871344001385284, 0.8893705212896308998, 0.000000000000000000 ) ) ;
#14147=VECTOR ( 'NONE', #11967, 1000.000000000000000 ) ;
#14150=EDGE_LOOP ( 'NONE', ( #6113, #13469, #1461, #8679 ) ) ;
#14151=CARTESIAN_POINT ( 'NONE',  ( 111.6227766016837961, 7.610970684806392799E-15, 7.000000000000000000 ) ) ;
#14164=AXIS2_PLACEMENT_3D ( 'NONE', #13268, #665, #4140 ) ;
#14165=DIRECTION ( 'NONE',  ( 0.1643989873053574580, -0.9863939238321436376, 0.000000000000000000 ) ) ;
#14182=EDGE_CURVE ( 'NONE', #7470, #13819, #2402, .T. ) ;
#14184=FACE_BOUND ( 'NONE', #8525, .T. ) ;
#14188=CARTESIAN_POINT ( 'NONE',  ( 19.25177984293775424, 7.759396820770413150, 7.000000000000006217 ) ) ;
#14199=ADVANCED_FACE ( 'NONE', ( #4477 ), #11533, .F. ) ;
#14203=CARTESIAN_POINT ( 'NONE',  ( 19.20634328910001543, -26.21503864878155099, 5.000000000000000000 ) ) ;
#14205=DIRECTION ( 'NONE',  ( 0.8893705212896308998, -0.4571871344001385284, 0.000000000000000000 ) ) ;
#14213=ORIENTED_EDGE ( 'NONE', *, *, #901, .F. ) ;
#14223=ORIENTED_EDGE ( 'NONE', *, *, #6823, .F. ) ;
#14235=DIRECTION ( 'NONE',  ( 1.000000000000000000, 0.000000000000000000, 0.000000000000000000 ) ) ;
#14248=DIRECTION ( 'NONE',  ( 0.000000000000000000, 0.000000000000000000, 1.000000000000000000 ) ) ;
#14257=DIRECTION ( 'NONE',  ( 0.000000000000000000, 0.000000000000000000, 1.000000000000000000 ) ) ;
#14260=ADVANCED_FACE ( 'NONE', ( #11760, #8445 ), #14067, .T. ) ;
#14266=ORIENTED_EDGE ( 'NONE', *, *, #3814, .T. ) ;
#14272=EDGE_CURVE ( 'NONE', #12669, #12714, #8223, .T. ) ;
#14275=ORIENTED_EDGE ( 'NONE', *, *, #3097, .T. ) ;
#14282=CARTESIAN_POINT ( 'NONE',  ( 62.65957446808508280, 26.91300136313512681, -8.169391093593850073 ) ) ;
#14284=DIRECTION ( 'NONE',  ( 1.000000000000000000, 0.000000000000000000, 0.000000000000000000 ) ) ;
#14286=ADVANCED_FACE ( 'NONE', ( #6152 ), #1238, .T. ) ;
#14299=VECTOR ( 'NONE', #8423, 1000.000000000000000 ) ;
#14300=AXIS2_PLACEMENT_3D ( 'NONE', #12411, #6581, #3124 ) ;
#14305=EDGE_LOOP ( 'NONE', ( #6147, #9294, #6504, #3594 ) ) ;
#14313=EDGE_CURVE ( 'NONE', #3242, #3993, #13944, .T. ) ;
#14326=ORIENTED_EDGE ( 'NONE', *, *, #12634, .T. ) ;
#14340=ORIENTED_EDGE ( 'NONE', *, *, #170, .F. ) ;
#14347=ADVANCED_FACE ( 'NONE', ( #3613 ), #4938, .T. ) ;
#14354=DIRECTION ( 'NONE',  ( -0.9863939238321437486, -0.1643989873053572359, 0.000000000000000000 ) ) ;
#14360=VERTEX_POINT ( 'NONE', #7154 ) ;
#14407=CARTESIAN_POINT ( 'NONE',  ( 101.6227766016837819, 5.204170427930421283E-15, 4.000000000000003553 ) ) ;
#14410=VECTOR ( 'NONE', #370, 1000.000000000000000 ) ;
#14427=CARTESIAN_POINT ( 'NONE',  ( -9.999999999999998224, 0.000000000000000000, -130.1575142076926852 ) ) ;
#14429=AXIS2_PLACEMENT_3D ( 'NONE', #3294, #13821, #4459 ) ;
#14434=ADVANCED_BREP_SHAPE_REPRESENTATION ( '', ( #13393, #1376 ), #2887 ) ;
#14437=AXIS2_PLACEMENT_3D ( 'NONE', #11677, #13999, #3399 ) ;
#14444=LINE ( 'NONE', #14282, #14299 ) ;
#14456=AXIS2_PLACEMENT_3D ( 'NONE', #14068, #1084, #3400 ) ;
#14457=CARTESIAN_POINT ( 'NONE',  ( 54.00962148274519592, 34.79915921274093193, 4.000000000000000000 ) ) ;
#14479=CIRCLE ( 'NONE', #6630, 20.00000000000000000 ) ;
#14481=EDGE_CURVE ( 'NONE', #11965, #5795, #12217, .T. ) ;
#14492=DIRECTION ( 'NONE',  ( -0.000000000000000000, -0.000000000000000000, -1.000000000000000000 ) ) ;
#14497=ORIENTED_EDGE ( 'NONE', *, *, #4012, .F. ) ;
#14503=DIRECTION ( 'NONE',  ( -0.000000000000000000, -0.000000000000000000, 1.000000000000000000 ) ) ;
#14504=DIRECTION ( 'NONE',  ( -0.000000000000000000, -0.000000000000000000, 1.000000000000000000 ) ) ;
#14513=CARTESIAN_POINT ( 'NONE',  ( 15.21482963846748504, 16.90833299098317610, 4.000000000000003553 ) ) ;
#14519=CYLINDRICAL_SURFACE ( 'NONE', #11833, 4.000000000000000000 ) ;
#14520=ORIENTED_EDGE ( 'NONE', *, *, #10696, .F. ) ;
#14522=DIRECTION ( 'NONE',  ( -0.000000000000000000, -0.000000000000000000, -1.000000000000000000 ) ) ;
#14530=VERTEX_POINT ( 'NONE', #4385 ) ;
#14550=CARTESIAN_POINT ( 'NONE',  ( 93.63799900313689761, -2.337932895214617002, 7.000000000000000000 ) ) ;
#14555=CARTESIAN_POINT ( 'NONE',  ( 93.63799900313688340, -2.337932895214617890, 7.000000000000000000 ) ) ;
#14576=CARTESIAN_POINT ( 'NONE',  ( 1.666666666666673624, 0.000000000000000000, 7.000000000000000000 ) ) ;
#14579=ORIENTED_EDGE ( 'NONE', *, *, #11356, .F. ) ;
#14599=CARTESIAN_POINT ( 'NONE',  ( 75.20570977803312473, 12.97982004111159959, -2.000000000000000888 ) ) ;
#14620=VECTOR ( 'NONE', #14503, 1000.000000000000000 ) ;
#14680=ORIENTED_EDGE ( 'NONE', *, *, #14005, .T. ) ;
#14682=( GEOMETRIC_REPRESENTATION_CONTEXT ( 3 ) GLOBAL_UNCERTAINTY_ASSIGNED_CONTEXT ( ( #7477 ) ) GLOBAL_UNIT_ASSIGNED_CONTEXT ( ( #3886, #5279, #8567 ) ) REPRESENTATION_CONTEXT ( 'NONE', 'WORKASPACE' ) );
#14684=CARTESIAN_POINT ( 'NONE',  ( 56.98919079003883326, 3.953582723775848962, 4.000000000000000000 ) ) ;
#14687=AXIS2_PLACEMENT_3D ( 'NONE', #8624, #7338, #9707 ) ;
#14695=EDGE_CURVE ( 'NONE', #2817, #6170, #4692, .T. ) ;
#14712=EDGE_CURVE ( 'NONE', #6698, #3271, #9429, .T. ) ;
#14715=DIRECTION ( 'NONE',  ( 0.000000000000000000, 0.000000000000000000, 1.000000000000000000 ) ) ;
#14738=VECTOR ( 'NONE', #12865, 1000.000000000000114 ) ;
#14743=DIRECTION ( 'NONE',  ( -0.4036950204470263204, 0.9148936170212770280, 0.000000000000000000 ) ) ;
#14745=CARTESIAN_POINT ( 'NONE',  ( 13.28797974610715116, -21.11867004231547540, 4.000000000000000000 ) ) ;
#14753=DIRECTION ( 'NONE',  ( -0.9148936170212769170, -0.4036950204470262649, 0.000000000000000000 ) ) ;
#14757=ORIENTED_EDGE ( 'NONE', *, *, #8807, .F. ) ;
#14758=ADVANCED_FACE ( 'NONE', ( #11877 ), #8420, .F. ) ;
#14766=CARTESIAN_POINT ( 'NONE',  ( 91.46153288930040048, 16.46030115554384565, 7.000000000000000000 ) ) ;
#14778=FACE_OUTER_BOUND ( 'NONE', #1636, .T. ) ;
#14792=VERTEX_POINT ( 'NONE', #1281 ) ;
#14795=VECTOR ( 'NONE', #1930, 1000.000000000000227 ) ;
#14806=AXIS2_PLACEMENT_3D ( 'NONE', #14407, #14492, #6405 ) ;
#14814=LINE ( 'NONE', #8960, #4122 ) ;
#14822=DIRECTION ( 'NONE',  ( -0.8893705212896292345, 0.4571871344001418036, 0.000000000000000000 ) ) ;
#14833=CARTESIAN_POINT ( 'NONE',  ( 13.78117670802322259, -24.07785181381190753, -2.000000000000000000 ) ) ;
#14839=EDGE_CURVE ( 'NONE', #11986, #4864, #1168, .T. ) ;
#14848=EDGE_LOOP ( 'NONE', ( #10626, #279, #8871, #7717 ) ) ;
#14849=VERTEX_POINT ( 'NONE', #4055 ) ;
#14850=ORIENTED_EDGE ( 'NONE', *, *, #11899, .F. ) ;
#14869=CIRCLE ( 'NONE', #7005, 1.999999999999998446 ) ;
#14870=AXIS2_PLACEMENT_3D ( 'NONE', #4489, #9326, #3255 ) ;
#14874=EDGE_CURVE ( 'NONE', #4008, #5666, #2748, .T. ) ;
#14889=DIRECTION ( 'NONE',  ( 1.000000000000000000, 0.000000000000000000, 0.000000000000000000 ) ) ;
#14890=CARTESIAN_POINT ( 'NONE',  ( 61.44848940674400239, 29.65768221419895667, 2.000000000000000000 ) ) ;
#14893=VECTOR ( 'NONE', #2835, 1000.000000000000114 ) ;
#14897=EDGE_LOOP ( 'NONE', ( #6802, #11733, #1668, #11363 ) ) ;
#14925=STYLED_ITEM ( 'NONE', ( #1572 ), #14434 ) ;
#14927=VECTOR ( 'NONE', #13752, 1000.000000000000000 ) ;
#14928=EDGE_LOOP ( 'NONE', ( #3795, #9613 ) ) ;
#14957=VERTEX_POINT ( 'NONE', #11342 ) ;
#14958=DIRECTION ( 'NONE',  ( -0.000000000000000000, -0.000000000000000000, 1.000000000000000000 ) ) ;
#14967=EDGE_LOOP ( 'NONE', ( #3950, #13385, #3561, #11300 ) ) ;
#14969=ORIENTED_EDGE ( 'NONE', *, *, #11356, .T. ) ;
#14985=DIRECTION ( 'NONE',  ( 0.000000000000000000, 0.000000000000000000, 1.000000000000000000 ) ) ;
#14987=EDGE_CURVE ( 'NONE', #14792, #1504, #4351, .T. ) ;
#14988=CARTESIAN_POINT ( 'NONE',  ( 59.43001430450886602, 34.23215029930534570, -2.000000000000000000 ) ) ;
#14999=PLANE ( 'NONE',  #3733 ) ;
#15004=EDGE_LOOP ( 'NONE', ( #13855, #774, #11616, #6447, #7070 ) ) ;
#15021=FACE_OUTER_BOUND ( 'NONE', #6672, .T. ) ;
#15022=ORIENTED_EDGE ( 'NONE', *, *, #8016, .F. ) ;
#15025=EDGE_CURVE ( 'NONE', #9696, #11269, #2046, .T. ) ;
#15049=CIRCLE ( 'NONE', #8397, 4.000000000000003553 ) ;
#15055=ORIENTED_EDGE ( 'NONE', *, *, #3097, .F. ) ;
#15061=CARTESIAN_POINT ( 'NONE',  ( 60.64109936584995353, 31.48746944824151583, -2.000000000000000000 ) ) ;
#15066=CARTESIAN_POINT ( 'NONE',  ( 14.27437366993929579, -27.03703358530833967, 5.000000000000000000 ) ) ;
#15068=ADVANCED_FACE ( 'NONE', ( #12422 ), #4441, .F. ) ;
#15071=VERTEX_POINT ( 'NONE', #9047 ) ;
#15072=ORIENTED_EDGE ( 'NONE', *, *, #2577, .F. ) ;
#15079=EDGE_CURVE ( 'NONE', #2255, #4549, #14814, .T. ) ;
#15082=AXIS2_PLACEMENT_3D ( 'NONE', #5246, #12300, #13533 ) ;
#15101=ORIENTED_EDGE ( 'NONE', *, *, #9963, .F. ) ;
#15115=ORIENTED_EDGE ( 'NONE', *, *, #2874, .F. ) ;
#15119=EDGE_CURVE ( 'NONE', #1742, #8861, #5111, .T. ) ;
#15147=EDGE_CURVE ( 'NONE', #5795, #2494, #6960, .T. ) ;
#15151=VECTOR ( 'NONE', #7796, 1000.000000000000000 ) ;
#15174=EDGE_CURVE ( 'NONE', #11965, #12266, #5958, .T. ) ;
#15178=CARTESIAN_POINT ( 'NONE',  ( 56.98919079003883326, 3.953582723775848962, 4.000000000000000000 ) ) ;
#15182=ORIENTED_EDGE ( 'NONE', *, *, #7156, .T. ) ;
#15185=CYLINDRICAL_SURFACE ( 'NONE', #13631, 4.000000000000003553 ) ;
#15190=CARTESIAN_POINT ( 'NONE',  ( 67.45386469005195806, 13.93318132202354676, -2.000000000000000888 ) ) ;
#15194=AXIS2_PLACEMENT_3D ( 'NONE', #9809, #6193, #4975 ) ;
#15195=DIRECTION ( 'NONE',  ( -0.000000000000000000, -0.000000000000000000, -1.000000000000000000 ) ) ;
#15198=ORIENTED_EDGE ( 'NONE', *, *, #901, .T. ) ;
#15199=CYLINDRICAL_SURFACE ( 'NONE', #11233, 2.000000000000003109 ) ;
#15259=COLOUR_RGB('Sky Blue',0.24,0.69,0.87);
#15260=FILL_AREA_STYLE_COLOUR('',#15259);
#15261=FILL_AREA_STYLE('',(#15260));
#15262=SURFACE_STYLE_FILL_AREA(#15261);
#15263=SURFACE_SIDE_STYLE('',(#15262));
#15264=SURFACE_STYLE_USAGE(.BOTH.,#15263);
#15265=PRESENTATION_STYLE_ASSIGNMENT((#15264));
ENDSEC;
END-ISO-10303-21;
